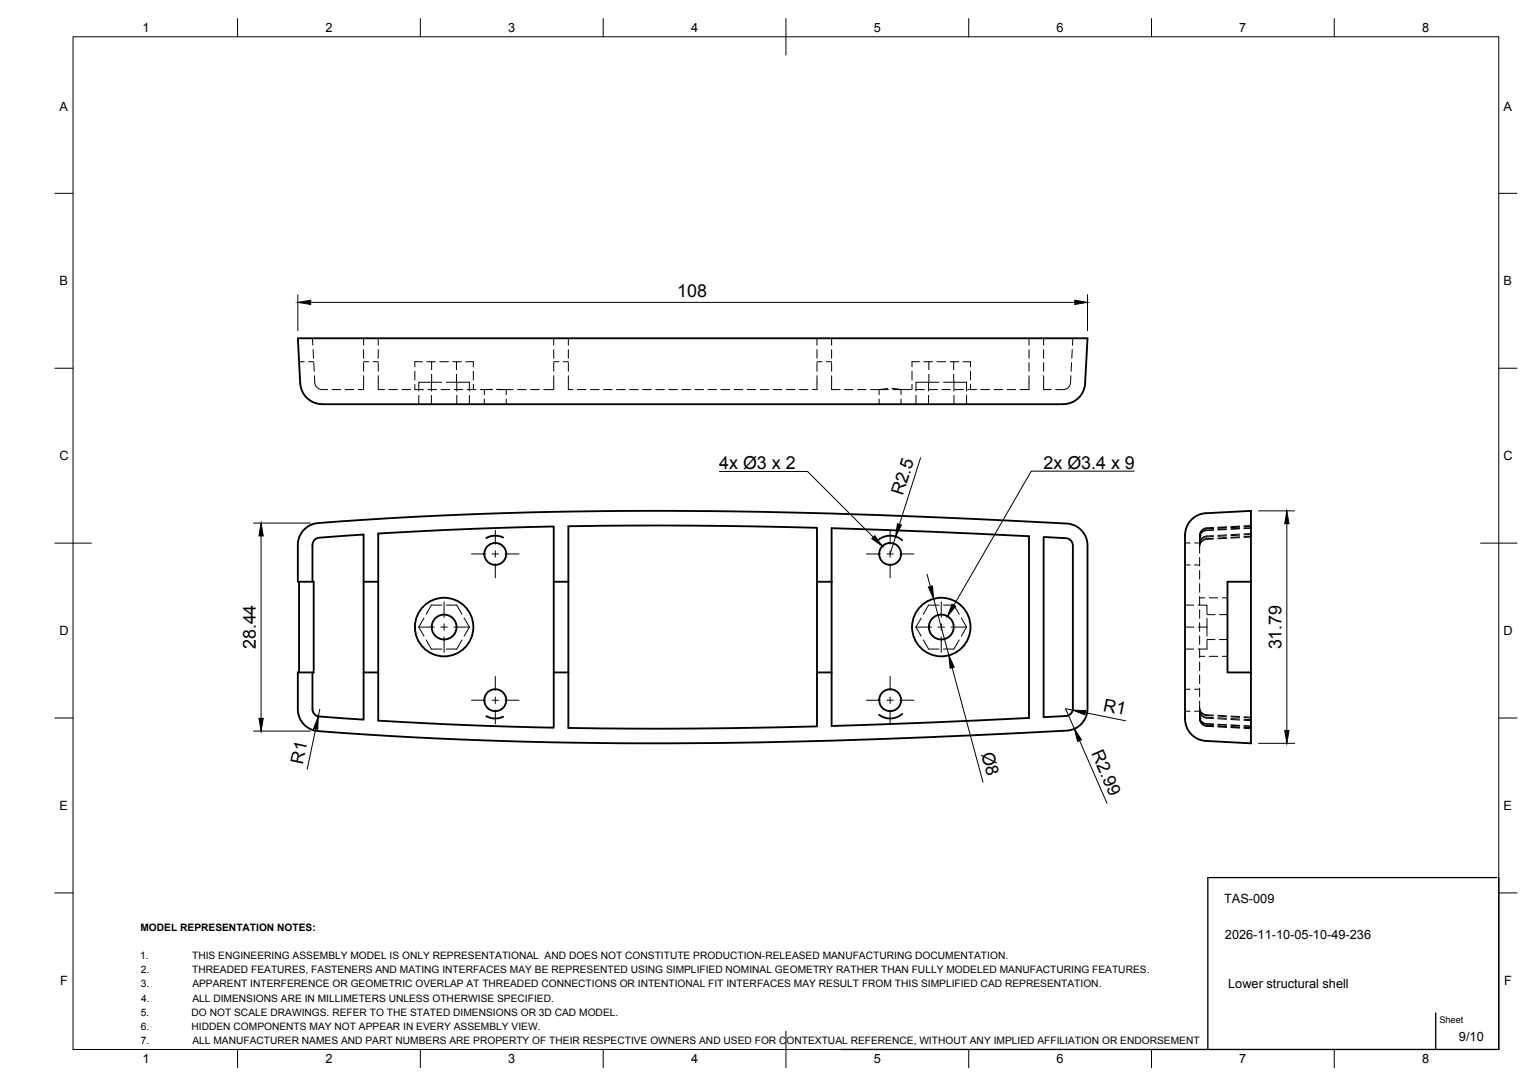
ISO-10303-21;
HEADER;
/* Generated by software containing ST-Developer
 * from STEP Tools, Inc. (www.steptools.com) 
 */

FILE_DESCRIPTION(
/* description */ (''),
/* implementation_level */ '2;1');

FILE_NAME(
/* name */ 'Lower structural shell.step',
/* time_stamp */ '2026-11-12T00:53:40-08:00',
/* author */ (''),
/* organization */ (''),
/* preprocessor_version */ 'ST-DEVELOPER v20.2',
/* originating_system */ 'Autodesk Translation Framework v15.17.0.0',
/* authorisation */ '');

FILE_SCHEMA (('AUTOMOTIVE_DESIGN { 1 0 10303 214 3 1 1 }'));
ENDSEC;

DATA;
#10=MECHANICAL_DESIGN_GEOMETRIC_PRESENTATION_REPRESENTATION('',(#576),#22129);
#84=SPHERICAL_SURFACE('',#9277,0.1);
#85=SPHERICAL_SURFACE('',#9280,0.0999999999999998);
#86=SPHERICAL_SURFACE('',#9284,0.0999999999999993);
#87=SPHERICAL_SURFACE('',#9288,0.1);
#88=SPHERICAL_SURFACE('',#9293,0.3);
#89=SPHERICAL_SURFACE('',#9297,0.3);
#90=SPHERICAL_SURFACE('',#9301,0.299999999999999);
#91=SPHERICAL_SURFACE('',#9306,0.3);
#124=B_SPLINE_SURFACE_WITH_KNOTS('',3,3,((#14410,#14411,#14412,#14413),
(#14414,#14415,#14416,#14417),(#14418,#14419,#14420,#14421),(#14422,#14423,
#14424,#14425),(#14426,#14427,#14428,#14429)),.UNSPECIFIED.,.F.,.F.,.F.,
(4,1,4),(4,4),(0.,0.571428571428571,1.),(1.0454440030657,3.44967454744645),
 .UNSPECIFIED.);
#125=B_SPLINE_SURFACE_WITH_KNOTS('',3,3,((#14502,#14503,#14504,#14505),
(#14506,#14507,#14508,#14509),(#14510,#14511,#14512,#14513),(#14514,#14515,
#14516,#14517),(#14518,#14519,#14520,#14521)),.UNSPECIFIED.,.F.,.F.,.F.,
(4,1,4),(4,4),(0.,0.571428571428571,1.),(7.24519303641511,9.95046872158573),
 .UNSPECIFIED.);
#126=B_SPLINE_SURFACE_WITH_KNOTS('',3,3,((#15443,#15444,#15445,#15446),
(#15447,#15448,#15449,#15450),(#15451,#15452,#15453,#15454),(#15455,#15456,
#15457,#15458)),.UNSPECIFIED.,.F.,.F.,.F.,(4,4),(4,4),(0.0705535719740953,
0.323522444336189),(0.0117434863834119,0.684857763552191),.UNSPECIFIED.);
#127=B_SPLINE_SURFACE_WITH_KNOTS('',3,3,((#15463,#15464,#15465,#15466),
(#15467,#15468,#15469,#15470),(#15471,#15472,#15473,#15474),(#15475,#15476,
#15477,#15478)),.UNSPECIFIED.,.F.,.F.,.F.,(4,4),(4,4),(0.0262419052680539,
0.0545428296147404),(0.0121538053864343,0.684980602226481),
 .UNSPECIFIED.);
#128=B_SPLINE_SURFACE_WITH_KNOTS('',3,3,((#15488,#15489,#15490,#15491),
(#15492,#15493,#15494,#15495),(#15496,#15497,#15498,#15499),(#15500,#15501,
#15502,#15503),(#15504,#15505,#15506,#15507)),.UNSPECIFIED.,.F.,.F.,.F.,
(4,1,4),(4,4),(0.,0.571428571428571,1.),(0.752061768057538,3.45733745322815),
 .UNSPECIFIED.);
#129=B_SPLINE_SURFACE_WITH_KNOTS('',3,3,((#15508,#15509,#15510,#15511),
(#15512,#15513,#15514,#15515),(#15516,#15517,#15518,#15519),(#15520,#15521,
#15522,#15523),(#15524,#15525,#15526,#15527)),.UNSPECIFIED.,.F.,.F.,.F.,
(4,1,4),(4,4),(0.,0.571428571428571,1.),(0.283259008618247,0.557056952888827),
 .UNSPECIFIED.);
#130=B_SPLINE_SURFACE_WITH_KNOTS('',3,3,((#15541,#15542,#15543,#15544),
(#15545,#15546,#15547,#15548),(#15549,#15550,#15551,#15552),(#15553,#15554,
#15555,#15556)),.UNSPECIFIED.,.F.,.F.,.F.,(4,4),(4,4),(0.67647755566375,
0.929446428026011),(0.0117434863436937,0.684857763580381),.UNSPECIFIED.);
#131=B_SPLINE_SURFACE_WITH_KNOTS('',3,3,((#15557,#15558,#15559,#15560),
(#15561,#15562,#15563,#15564),(#15565,#15566,#15567,#15568),(#15569,#15570,
#15571,#15572)),.UNSPECIFIED.,.F.,.F.,.F.,(4,4),(4,4),(0.945457170385156,
0.973758094731946),(0.0121538053598088,0.684980602226481),.UNSPECIFIED.);
#132=B_SPLINE_SURFACE_WITH_KNOTS('',3,3,((#15656,#15657,#15658,#15659),
(#15660,#15661,#15662,#15663),(#15664,#15665,#15666,#15667),(#15668,#15669,
#15670,#15671)),.UNSPECIFIED.,.F.,.F.,.F.,(4,4),(4,4),(0.341142793678372,
0.658675488550287),(0.0116221239297273,0.684255166525269),.UNSPECIFIED.);
#133=B_SPLINE_SURFACE_WITH_KNOTS('',3,3,((#15676,#15677,#15678,#15679),
(#15680,#15681,#15682,#15683),(#15684,#15685,#15686,#15687),(#15688,#15689,
#15690,#15691),(#15692,#15693,#15694,#15695)),.UNSPECIFIED.,.F.,.F.,.F.,
(4,1,4),(4,4),(0.,0.571428571428571,1.),(3.65450559744172,7.0548588409572),
 .UNSPECIFIED.);
#134=B_SPLINE_SURFACE_WITH_KNOTS('',3,3,((#15705,#15706,#15707,#15708),
(#15709,#15710,#15711,#15712),(#15713,#15714,#15715,#15716),(#15717,#15718,
#15719,#15720),(#15721,#15722,#15723,#15724)),.UNSPECIFIED.,.F.,.F.,.F.,
(4,1,4),(4,4),(0.,0.571428571428571,1.),(3.64767164868607,7.04802489220155),
 .UNSPECIFIED.);
#135=B_SPLINE_SURFACE_WITH_KNOTS('',3,3,((#15729,#15730,#15731,#15732),
(#15733,#15734,#15735,#15736),(#15737,#15738,#15739,#15740),(#15741,#15742,
#15743,#15744)),.UNSPECIFIED.,.F.,.F.,.F.,(4,4),(4,4),(0.341324511449716,
0.658857206321627),(0.0116221214776208,0.684255166525269),.UNSPECIFIED.);
#136=B_SPLINE_SURFACE_WITH_KNOTS('',3,3,((#15789,#15790,#15791,#15792),
(#15793,#15794,#15795,#15796),(#15797,#15798,#15799,#15800),(#15801,#15802,
#15803,#15804)),.UNSPECIFIED.,.F.,.F.,.F.,(4,4),(4,4),(0.676316266718331,
0.901708040522105),(0.0117102006467275,0.68495201331719),.UNSPECIFIED.);
#137=B_SPLINE_SURFACE_WITH_KNOTS('',3,3,((#15809,#15810,#15811,#15812),
(#15813,#15814,#15815,#15816),(#15817,#15818,#15819,#15820),(#15821,#15822,
#15823,#15824),(#15825,#15826,#15827,#15828)),.UNSPECIFIED.,.F.,.F.,.F.,
(4,1,4),(4,4),(0.,0.571428571428571,1.),(7.25285594219682,9.65708648657758),
 .UNSPECIFIED.);
#138=B_SPLINE_SURFACE_WITH_KNOTS('',3,3,((#15838,#15839,#15840,#15841),
(#15842,#15843,#15844,#15845),(#15846,#15847,#15848,#15849),(#15850,#15851,
#15852,#15853)),.UNSPECIFIED.,.F.,.F.,.F.,(4,4),(4,4),(0.0982919594778951,
0.323683733281714),(0.0117102006467272,0.68495201331719),.UNSPECIFIED.);
#139=B_SPLINE_SURFACE_WITH_KNOTS('',3,3,((#15928,#15929,#15930,#15931),
(#15932,#15933,#15934,#15935),(#15936,#15937,#15938,#15939),(#15940,#15941,
#15942,#15943)),.UNSPECIFIED.,.F.,.F.,.F.,(4,4),(4,4),(0.917922863855343,
0.974411608827007),(0.0122403473423911,0.685344304754238),.UNSPECIFIED.);
#140=B_SPLINE_SURFACE_WITH_KNOTS('',3,3,((#15953,#15954,#15955,#15956),
(#15957,#15958,#15959,#15960),(#15961,#15962,#15963,#15964),(#15965,#15966,
#15967,#15968),(#15969,#15970,#15971,#15972)),.UNSPECIFIED.,.F.,.F.,.F.,
(4,1,4),(4,4),(0.,0.571428571428571,1.),(9.85085636625011,10.4271318523291),
 .UNSPECIFIED.);
#141=B_SPLINE_SURFACE_WITH_KNOTS('',3,3,((#15986,#15987,#15988,#15989),
(#15990,#15991,#15992,#15993),(#15994,#15995,#15996,#15997),(#15998,#15999,
#16000,#16001)),.UNSPECIFIED.,.F.,.F.,.F.,(4,4),(4,4),(0.025588391172993,
0.0820771361446569),(0.0122403473423911,0.685344304754238),
 .UNSPECIFIED.);
#142=B_SPLINE_SURFACE_WITH_KNOTS('',3,3,((#16011,#16012,#16013,#16014),
(#16015,#16016,#16017,#16018),(#16019,#16020,#16021,#16022),(#16023,#16024,
#16025,#16026),(#16027,#16028,#16029,#16030)),.UNSPECIFIED.,.F.,.F.,.F.,
(4,1,4),(4,4),(0.,0.571428571428571,1.),(0.27539863731415,0.851674123393175),
 .UNSPECIFIED.);
#143=B_SPLINE_SURFACE_WITH_KNOTS('',3,3,((#16044,#16045,#16046,#16047),
(#16048,#16049,#16050,#16051),(#16052,#16053,#16054,#16055),(#16056,#16057,
#16058,#16059),(#16060,#16061,#16062,#16063)),.UNSPECIFIED.,.F.,.F.,.F.,
(4,1,4),(4,4),(0.,0.571428571428571,1.),(0.00944995813270487,0.618489359031386),
 .UNSPECIFIED.);
#144=B_SPLINE_SURFACE_WITH_KNOTS('',3,3,((#16070,#16071,#16072,#16073),
(#16074,#16075,#16076,#16077),(#16078,#16079,#16080,#16081),(#16082,#16083,
#16084,#16085),(#16086,#16087,#16088,#16089)),.UNSPECIFIED.,.F.,.F.,.F.,
(4,1,4),(4,4),(0.,0.571428571428571,1.),(0.00908570715245136,0.618164468641375),
 .UNSPECIFIED.);
#145=B_SPLINE_SURFACE_WITH_KNOTS('',3,3,((#16094,#16095,#16096,#16097),
(#16098,#16099,#16100,#16101),(#16102,#16103,#16104,#16105),(#16106,#16107,
#16108,#16109),(#16110,#16111,#16112,#16113)),.UNSPECIFIED.,.F.,.F.,.F.,
(4,1,4),(4,4),(0.,0.571428571428571,1.),(0.0091183540525243,0.618164468641375),
 .UNSPECIFIED.);
#146=B_SPLINE_SURFACE_WITH_KNOTS('',3,3,((#16118,#16119,#16120,#16121),
(#16122,#16123,#16124,#16125),(#16126,#16127,#16128,#16129),(#16130,#16131,
#16132,#16133),(#16134,#16135,#16136,#16137)),.UNSPECIFIED.,.F.,.F.,.F.,
(4,1,4),(4,4),(0.,0.571428571428571,1.),(10.1454735367545,10.419271481025),
 .UNSPECIFIED.);
#147=B_SPLINE_SURFACE_WITH_KNOTS('',3,3,((#16138,#16139,#16140,#16141),
(#16142,#16143,#16144,#16145),(#16146,#16147,#16148,#16149),(#16150,#16151,
#16152,#16153),(#16154,#16155,#16156,#16157)),.UNSPECIFIED.,.F.,.F.,.F.,
(4,1,4),(4,4),(0.,0.571428571428571,1.),(0.0094045468285345,0.618489359031386),
 .UNSPECIFIED.);
#148=B_SPLINE_SURFACE_WITH_KNOTS('',3,3,((#16183,#16184,#16185,#16186),
(#16187,#16188,#16189,#16190),(#16191,#16192,#16193,#16194),(#16195,#16196,
#16197,#16198),(#16199,#16200,#16201,#16202)),.UNSPECIFIED.,.F.,.F.,.F.,
(4,1,4),(4,4),(0.,0.571428571428571,1.),(-0.00535061636073277,0.618489359031386),
 .UNSPECIFIED.);
#149=B_SPLINE_SURFACE_WITH_KNOTS('',3,3,((#16221,#16222,#16223,#16224,#16225),
(#16226,#16227,#16228,#16229,#16230),(#16231,#16232,#16233,#16234,#16235),
(#16236,#16237,#16238,#16239,#16240),(#16241,#16242,#16243,#16244,#16245)),
 .UNSPECIFIED.,.F.,.F.,.F.,(4,1,4),(4,1,4),(0.,0.571428571428571,1.),(0.283259008618247,
4.63063308449434,10.4271318523291),.UNSPECIFIED.);
#150=B_SPLINE_SURFACE_WITH_KNOTS('',3,3,((#16256,#16257,#16258,#16259),
(#16260,#16261,#16262,#16263),(#16264,#16265,#16266,#16267),(#16268,#16269,
#16270,#16271),(#16272,#16273,#16274,#16275)),.UNSPECIFIED.,.F.,.F.,.F.,
(4,1,4),(4,4),(0.,0.571428571428571,1.),(-0.00578978989683084,0.618164468641375),
 .UNSPECIFIED.);
#151=B_SPLINE_SURFACE_WITH_KNOTS('',3,3,((#16284,#16285,#16286,#16287),
(#16288,#16289,#16290,#16291),(#16292,#16293,#16294,#16295),(#16296,#16297,
#16298,#16299),(#16300,#16301,#16302,#16303)),.UNSPECIFIED.,.F.,.F.,.F.,
(4,1,4),(4,4),(0.,0.571428571428571,1.),(-0.00569189159989896,0.618164468641375),
 .UNSPECIFIED.);
#152=B_SPLINE_SURFACE_WITH_KNOTS('',3,3,((#16312,#16313,#16314,#16315,#16316),
(#16317,#16318,#16319,#16320,#16321),(#16322,#16323,#16324,#16325,#16326),
(#16327,#16328,#16329,#16330,#16331),(#16332,#16333,#16334,#16335,#16336)),
 .UNSPECIFIED.,.F.,.F.,.F.,(4,1,4),(4,1,4),(0.,0.571428571428571,1.),(0.27539863731415,
4.62277271319024,10.419271481025),.UNSPECIFIED.);
#153=B_SPLINE_SURFACE_WITH_KNOTS('',3,3,((#16347,#16348,#16349,#16350),
(#16351,#16352,#16353,#16354),(#16355,#16356,#16357,#16358),(#16359,#16360,
#16361,#16362),(#16363,#16364,#16365,#16366)),.UNSPECIFIED.,.F.,.F.,.F.,
(4,1,4),(4,4),(0.,0.571428571428571,1.),(-0.0054868135546625,0.618489359031386),
 .UNSPECIFIED.);
#154=B_SPLINE_SURFACE_WITH_KNOTS('',3,3,((#16375,#16376,#16377,#16378),
(#16379,#16380,#16381,#16382),(#16383,#16384,#16385,#16386),(#16387,#16388,
#16389,#16390)),.UNSPECIFIED.,.F.,.F.,.F.,(4,4),(4,4),(0.026239262514127,
0.974414173651419),(0.,0.685344304754238),.UNSPECIFIED.);
#155=B_SPLINE_SURFACE_WITH_KNOTS('',3,3,((#16393,#16394,#16395,#16396),
(#16397,#16398,#16399,#16400),(#16401,#16402,#16403,#16404),(#16405,#16406,
#16407,#16408)),.UNSPECIFIED.,.F.,.F.,.F.,(4,4),(4,4),(0.0255858263485814,
0.973760737485873),(0.,0.685344304754238),.UNSPECIFIED.);
#272=B_SPLINE_CURVE_WITH_KNOTS('',3,(#14309,#14310,#14311,#14312,#14313,
#14314,#14315,#14316,#14317,#14318,#14319,#14320,#14321,#14322,#14323,#14324,
#14325,#14326,#14327,#14328,#14329,#14330,#14331,#14332),.UNSPECIFIED.,
 .F.,.F.,(4,2,2,2,2,2,2,2,2,2,2,4),(-0.337265338267783,-0.250544943628509,
-0.208272806508042,-0.186542211788094,-0.176382978682897,-0.170925844043069,
-0.16639450677335,-0.161077381235501,-0.15182241135393,-0.115009181549223,
-0.030206004227969,0.),.UNSPECIFIED.);
#273=B_SPLINE_CURVE_WITH_KNOTS('',3,(#14337,#14338,#14339,#14340,#14341,
#14342,#14343,#14344,#14345,#14346,#14347,#14348,#14349,#14350,#14351,#14352,
#14353,#14354,#14355,#14356),.UNSPECIFIED.,.F.,.F.,(4,2,2,2,2,2,2,2,2,4),
(-0.240982594686416,-0.16829976149504,-0.141836598208813,-0.129116059226128,
-0.121962912034391,-0.115857591426886,-0.108506552485159,-0.0948769875819265,
-0.0364654790774683,0.),.UNSPECIFIED.);
#274=B_SPLINE_CURVE_WITH_KNOTS('',3,(#14361,#14362,#14363,#14364,#14365,
#14366,#14367,#14368,#14369,#14370,#14371,#14372,#14373,#14374,#14375,#14376,
#14377,#14378,#14379,#14380),.UNSPECIFIED.,.F.,.F.,(4,2,2,2,2,2,2,2,2,4),
(-0.240981214998207,-0.168303541671295,-0.141841407502325,-0.129121097580905,
-0.121968013294536,-0.115862708924237,-0.108511643765797,-0.0948818976588229,
-0.0364681276985956,0.),.UNSPECIFIED.);
#275=B_SPLINE_CURVE_WITH_KNOTS('',3,(#14385,#14386,#14387,#14388,#14389,
#14390,#14391,#14392,#14393,#14394,#14395,#14396,#14397,#14398,#14399,#14400,
#14401,#14402,#14403,#14404,#14405,#14406,#14407,#14408),.UNSPECIFIED.,
 .F.,.F.,(4,2,2,2,2,2,2,2,2,2,2,4),(-0.337269388373684,-0.250545316912909,
-0.208282401844766,-0.186554569827561,-0.176396213396297,-0.17093921790305,
-0.16640782243471,-0.161090427650893,-0.151834477986603,-0.115010808423941,
-0.0302102096065556,0.),.UNSPECIFIED.);
#276=B_SPLINE_CURVE_WITH_KNOTS('',3,(#14431,#14432,#14433,#14434),
 .UNSPECIFIED.,.F.,.F.,(4,4),(1.0454440030657,2.52465537163019),
 .UNSPECIFIED.);
#277=B_SPLINE_CURVE_WITH_KNOTS('',3,(#14436,#14437,#14438,#14439,#14440,
#14441,#14442,#14443,#14444,#14445,#14446,#14447,#14448,#14449,#14450,#14451,
#14452,#14453,#14454,#14455,#14456,#14457,#14458,#14459,#14460,#14461,#14462,
#14463),.UNSPECIFIED.,.F.,.F.,(4,3,3,3,3,3,3,3,3,4),(-0.152193408756968,
-0.128427023368412,-0.115107736263918,-0.0911810900745799,-0.0780377802127556,
-0.0652031397886901,-0.0414031558437525,-0.0389949527774582,-0.0152076153333754,
0.),.UNSPECIFIED.);
#278=B_SPLINE_CURVE_WITH_KNOTS('',3,(#14465,#14466,#14467,#14468),
 .UNSPECIFIED.,.F.,.F.,(4,4),(-3.44967454744645,-1.05170160817356),
 .UNSPECIFIED.);
#279=B_SPLINE_CURVE_WITH_KNOTS('',3,(#14470,#14471,#14472,#14473,#14474,
#14475,#14476,#14477,#14478,#14479,#14480,#14481,#14482,#14483,#14484,#14485,
#14486,#14487,#14488,#14489,#14490,#14491,#14492,#14493,#14494,#14495,#14496,
#14497),.UNSPECIFIED.,.F.,.F.,(4,3,3,3,3,3,3,3,3,4),(-0.152278960443096,
-0.128503570101575,-0.115218572146868,-0.09145408274965,-0.0870214650669139,
-0.0781562978024333,-0.0542566895399357,-0.03908030849237,-0.0153296112319379,
0.),.UNSPECIFIED.);
#280=B_SPLINE_CURVE_WITH_KNOTS('',3,(#14498,#14499,#14500,#14501),
 .UNSPECIFIED.,.F.,.F.,(4,4),(2.75501813708031,3.4476340663212),
 .UNSPECIFIED.);
#281=B_SPLINE_CURVE_WITH_KNOTS('',3,(#14523,#14524,#14525,#14526),
 .UNSPECIFIED.,.F.,.F.,(4,4),(7.24810383506675,7.89761558728778),
 .UNSPECIFIED.);
#282=B_SPLINE_CURVE_WITH_KNOTS('',3,(#14528,#14529,#14530,#14531,#14532,
#14533,#14534,#14535,#14536,#14537,#14538,#14539,#14540,#14541,#14542,#14543,
#14544,#14545,#14546,#14547,#14548,#14549,#14550,#14551,#14552,#14553,#14554,
#14555),.UNSPECIFIED.,.F.,.F.,(4,3,3,3,3,3,3,3,3,4),(-0.152278869104567,
-0.128548794904564,-0.115192257893812,-0.0912773536606376,-0.0781090575823055,
-0.0652724057916263,-0.0414819581560496,-0.0390493575290778,-0.015259721743698,
0.),.UNSPECIFIED.);
#283=B_SPLINE_CURVE_WITH_KNOTS('',3,(#14557,#14558,#14559,#14560),
 .UNSPECIFIED.,.F.,.F.,(4,4),(-9.94532343034734,-7.24519303641511),
 .UNSPECIFIED.);
#284=B_SPLINE_CURVE_WITH_KNOTS('',3,(#14562,#14563,#14564,#14565,#14566,
#14567,#14568,#14569,#14570,#14571,#14572,#14573,#14574,#14575,#14576,#14577,
#14578,#14579,#14580,#14581,#14582,#14583,#14584,#14585,#14586,#14587,#14588,
#14589),.UNSPECIFIED.,.F.,.F.,(4,3,3,3,3,3,3,3,3,4),(-0.152181623618259,
-0.128410404494075,-0.115248188224843,-0.0914746846046984,-0.0869904866333268,
-0.0783028696190655,-0.0543945376065823,-0.0391651209697638,-0.0153884182770307,
0.),.UNSPECIFIED.);
#285=B_SPLINE_CURVE_WITH_KNOTS('',3,(#14590,#14591,#14592,#14593),
 .UNSPECIFIED.,.F.,.F.,(4,4),(8.21380824320284,9.95046871680089),
 .UNSPECIFIED.);
#286=B_SPLINE_CURVE_WITH_KNOTS('',3,(#14596,#14597,#14598,#14599),
 .UNSPECIFIED.,.F.,.F.,(4,4),(2.80491490332713,3.45442665446657),
 .UNSPECIFIED.);
#287=B_SPLINE_CURVE_WITH_KNOTS('',3,(#14603,#14604,#14605,#14606),
 .UNSPECIFIED.,.F.,.F.,(4,4),(0.752061768057538,2.48872224644044),
 .UNSPECIFIED.);
#288=B_SPLINE_CURVE_WITH_KNOTS('',3,(#14814,#14815,#14816,#14817,#14818,
#14819),.UNSPECIFIED.,.F.,.F.,(4,2,4),(-0.606700505977711,-0.303383635264422,
-0.000339350725729326),.UNSPECIFIED.);
#289=B_SPLINE_CURVE_WITH_KNOTS('',3,(#14820,#14821,#14822,#14823,#14824,
#14825,#14826,#14827,#14828,#14829,#14830,#14831,#14832,#14833,#14834,#14835,
#14836,#14837,#14838,#14839,#14840,#14841,#14842,#14843,#14844,#14845,#14846,
#14847),.UNSPECIFIED.,.F.,.F.,(4,3,3,3,3,3,3,3,3,4),(-0.152173579228948,
-0.128423230539522,-0.115115104157663,-0.0911927259648815,-0.0780672068328041,
-0.0652082609452843,-0.0414117413801899,-0.0390174000215468,-0.0152300060615686,
0.),.UNSPECIFIED.);
#290=B_SPLINE_CURVE_WITH_KNOTS('',3,(#14848,#14849,#14850,#14851,#14852,
#14853),.UNSPECIFIED.,.F.,.F.,(4,2,4),(-0.606471894652381,-0.303383500305553,
-0.00011071898471493),.UNSPECIFIED.);
#291=B_SPLINE_CURVE_WITH_KNOTS('',3,(#14857,#14858,#14859,#14860,#14861,
#14862),.UNSPECIFIED.,.F.,.F.,(4,2,4),(-0.606240625011114,-0.303433113375332,
-0.00010938105916114),.UNSPECIFIED.);
#292=B_SPLINE_CURVE_WITH_KNOTS('',3,(#14864,#14865,#14866,#14867,#14868,
#14869,#14870,#14871,#14872,#14873,#14874,#14875,#14876,#14877,#14878,#14879,
#14880,#14881,#14882,#14883,#14884,#14885,#14886,#14887,#14888,#14889,#14890,
#14891),.UNSPECIFIED.,.F.,.F.,(4,3,3,3,3,3,3,3,3,4),(-0.152281454644235,
-0.128508102092242,-0.115234945630277,-0.0914677943501604,-0.0870276017853555,
-0.0781846052914712,-0.0542821334115454,-0.0390966859411886,-0.0153419673568312,
0.),.UNSPECIFIED.);
#293=B_SPLINE_CURVE_WITH_KNOTS('',3,(#14893,#14894,#14895,#14896,#14897,
#14898),.UNSPECIFIED.,.F.,.F.,(4,2,4),(-0.606758573154242,-0.303433157101101,
-0.000627306481538803),.UNSPECIFIED.);
#294=B_SPLINE_CURVE_WITH_KNOTS('',3,(#14904,#14905,#14906,#14907,#14908,
#14909),.UNSPECIFIED.,.F.,.F.,(4,2,4),(-0.60617382748,-0.303436117212405,
-7.2700296824213E-5),.UNSPECIFIED.);
#295=B_SPLINE_CURVE_WITH_KNOTS('',3,(#14911,#14912,#14913,#14914,#14915,
#14916,#14917,#14918,#14919,#14920,#14921,#14922,#14923,#14924,#14925,#14926,
#14927,#14928,#14929,#14930,#14931,#14932,#14933,#14934,#14935,#14936,#14937,
#14938),.UNSPECIFIED.,.F.,.F.,(4,3,3,3,3,3,3,3,3,4),(-0.152282154327755,
-0.128558036203745,-0.115201429639692,-0.0912891813973639,-0.0781219052297615,
-0.065279687589213,-0.0414913146723999,-0.0390591331507366,-0.0152683745546824,
0.),.UNSPECIFIED.);
#296=B_SPLINE_CURVE_WITH_KNOTS('',3,(#14942,#14943,#14944,#14945,#14946,
#14947,#14948,#14949,#14950,#14951,#14952,#14953,#14954,#14955,#14956,#14957,
#14958,#14959,#14960,#14961,#14962,#14963,#14964,#14965,#14966,#14967,#14968,
#14969),.UNSPECIFIED.,.F.,.F.,(4,3,3,3,3,3,3,3,3,4),(-0.152283066055976,
-0.128508717930245,-0.115216472798554,-0.091451700383826,-0.087022506454752,
-0.0781485278686168,-0.0542483994686567,-0.0390758108455304,-0.0153274175274101,
0.),.UNSPECIFIED.);
#297=B_SPLINE_CURVE_WITH_KNOTS('',3,(#14971,#14972,#14973,#14974,#14975,
#14976),.UNSPECIFIED.,.F.,.F.,(4,2,4),(-0.606800264911061,-0.303436147592132,
-0.000699137727853738),.UNSPECIFIED.);
#298=B_SPLINE_CURVE_WITH_KNOTS('',3,(#14981,#14982,#14983,#14984,#14985,
#14986),.UNSPECIFIED.,.F.,.F.,(4,2,4),(-0.606915279655722,-0.30363236403835,
-0.000516487074480598),.UNSPECIFIED.);
#299=B_SPLINE_CURVE_WITH_KNOTS('',3,(#14990,#14991,#14992,#14993,#14994,
#14995,#14996,#14997,#14998,#14999,#15000,#15001,#15002,#15003,#15004,#15005,
#15006,#15007,#15008,#15009,#15010,#15011,#15012,#15013,#15014,#15015,#15016,
#15017),.UNSPECIFIED.,.F.,.F.,(4,3,3,3,3,3,3,3,3,4),(-0.152205325335401,
-0.128433618138404,-0.115304790388008,-0.091527299141506,-0.0870178586418932,
-0.0783866443643876,-0.0544751548276533,-0.0392137310602028,-0.0154203878854647,
0.),.UNSPECIFIED.);
#300=B_SPLINE_CURVE_WITH_KNOTS('',3,(#15019,#15020,#15021,#15022,#15023,
#15024),.UNSPECIFIED.,.F.,.F.,(4,2,4),(-0.606752424187958,-0.303632696349781,
-0.000353591088346872),.UNSPECIFIED.);
#301=B_SPLINE_CURVE_WITH_KNOTS('',3,(#15030,#15031,#15032,#15033),
 .UNSPECIFIED.,.F.,.F.,(4,4),(0.0116023361771303,0.618489359031386),
 .UNSPECIFIED.);
#302=B_SPLINE_CURVE_WITH_KNOTS('',3,(#15037,#15038,#15039,#15040),
 .UNSPECIFIED.,.F.,.F.,(4,4),(-0.618489359031386,-0.01160233617713),
 .UNSPECIFIED.);
#303=B_SPLINE_CURVE_WITH_KNOTS('',3,(#15043,#15044,#15045,#15046),
 .UNSPECIFIED.,.F.,.F.,(4,4),(7.01593971618694,9.71770560667459),
 .UNSPECIFIED.);
#304=B_SPLINE_CURVE_WITH_KNOTS('',3,(#15047,#15048,#15049,#15050),
 .UNSPECIFIED.,.F.,.F.,(4,4),(0.505945342046796,3.20718651982575),
 .UNSPECIFIED.);
#305=B_SPLINE_CURVE_WITH_KNOTS('',3,(#15053,#15054,#15055,#15056,#15057,
#15058,#15059),.UNSPECIFIED.,.F.,.F.,(4,3,4),(3.40717417387402,5.11170895874517,
6.80746068626633),.UNSPECIFIED.);
#306=B_SPLINE_CURVE_WITH_KNOTS('',3,(#15062,#15063,#15064,#15065),
 .UNSPECIFIED.,.F.,.F.,(4,4),(7.00766573366377,9.41198845520559),
 .UNSPECIFIED.);
#307=B_SPLINE_CURVE_WITH_KNOTS('',3,(#15069,#15070,#15071,#15072),
 .UNSPECIFIED.,.F.,.F.,(4,4),(9.61248784142317,10.2217363065808),
 .UNSPECIFIED.);
#308=B_SPLINE_CURVE_WITH_KNOTS('',3,(#15073,#15074,#15075,#15076,#15077,
#15078,#15079,#15080,#15081,#15082,#15083,#15084,#15085,#15086,#15087,#15088,
#15089,#15090,#15091,#15092,#15093,#15094,#15095,#15096,#15097,#15098,#15099,
#15100),.UNSPECIFIED.,.F.,.F.,(4,3,3,3,3,3,3,3,3,4),(0.,0.0238103109064959,
0.0390781362249314,0.0628635086275546,0.0641230352384255,0.0780643700703951,
0.101962174814111,0.113803522271848,0.137549611554782,0.149564734365165),
 .UNSPECIFIED.);
#309=B_SPLINE_CURVE_WITH_KNOTS('',3,(#15104,#15105,#15106,#15107,#15108,
#15109,#15110,#15111,#15112,#15113,#15114,#15115,#15116,#15117,#15118,#15119,
#15120,#15121,#15122,#15123,#15124,#15125,#15126,#15127,#15128,#15129,#15130,
#15131,#15132,#15133,#15134),.UNSPECIFIED.,.F.,.F.,(4,3,3,3,3,3,3,3,3,3,
4),(0.,0.0535521515156599,0.107729685495911,0.117233338918226,0.171447998942947,
0.1923696899792,0.234191611538245,0.288659693466396,0.341410301570312,0.395549383747909,
0.448696573746633),.UNSPECIFIED.);
#310=B_SPLINE_CURVE_WITH_KNOTS('',3,(#15136,#15137,#15138,#15139),
 .UNSPECIFIED.,.F.,.F.,(4,4),(0.0255858263485814,0.973760737485873),
 .UNSPECIFIED.);
#311=B_SPLINE_CURVE_WITH_KNOTS('',3,(#15141,#15142,#15143,#15144,#15145,
#15146,#15147,#15148,#15149,#15150,#15151,#15152,#15153,#15154,#15155,#15156,
#15157,#15158,#15159,#15160,#15161,#15162,#15163,#15164,#15165,#15166,#15167,
#15168,#15169,#15170,#15171),.UNSPECIFIED.,.F.,.F.,(4,3,3,3,3,3,3,3,3,3,
4),(0.,0.0535144560117858,0.107726856902975,0.117300577410231,0.171517675930231,
0.195438847090422,0.234297456941738,0.289665153342662,0.345032849743585,
0.40043206955427,0.455831289364955),.UNSPECIFIED.);
#312=B_SPLINE_CURVE_WITH_KNOTS('',3,(#15175,#15176,#15177,#15178,#15179,
#15180,#15181,#15182,#15183,#15184,#15185,#15186,#15187,#15188,#15189,#15190,
#15191,#15192,#15193,#15194,#15195,#15196,#15197,#15198,#15199,#15200,#15201,
#15202,#15203,#15204,#15205),.UNSPECIFIED.,.F.,.F.,(4,3,3,3,3,3,3,3,3,3,
4),(0.,0.053505543180391,0.107714168832353,0.117253997025819,0.171473395203321,
0.195418854185489,0.234223199196375,0.289607016015183,0.344990832833991,
0.400409777473312,0.455828722112633),.UNSPECIFIED.);
#313=B_SPLINE_CURVE_WITH_KNOTS('',3,(#15207,#15208,#15209,#15210),
 .UNSPECIFIED.,.F.,.F.,(4,4),(0.0262392625141271,0.974414173651419),
 .UNSPECIFIED.);
#314=B_SPLINE_CURVE_WITH_KNOTS('',3,(#15212,#15213,#15214,#15215,#15216,
#15217,#15218,#15219,#15220,#15221,#15222,#15223,#15224,#15225,#15226,#15227,
#15228,#15229,#15230,#15231,#15232,#15233,#15234,#15235,#15236,#15237,#15238,
#15239,#15240,#15241,#15242),.UNSPECIFIED.,.F.,.F.,(4,3,3,3,3,3,3,3,3,3,
4),(0.,0.0535648734523888,0.107747221190676,0.117299947751206,0.171510987106922,
0.192397607227928,0.234296687348373,0.288768001369001,0.341469499352622,
0.395597672314973,0.448700135162036),.UNSPECIFIED.);
#315=B_SPLINE_CURVE_WITH_KNOTS('',3,(#15245,#15246,#15247,#15248,#15249,
#15250,#15251,#15252,#15253,#15254,#15255,#15256,#15257,#15258,#15259,#15260,
#15261,#15262,#15263,#15264,#15265,#15266,#15267,#15268,#15269),
 .UNSPECIFIED.,.F.,.F.,(4,3,3,3,3,3,3,3,4),(0.,0.0238141989470671,0.0391004231578824,
0.0641320992313133,0.0780996136084711,0.101998806889826,0.113823260594808,
0.137564745199532,0.149565921982294),.UNSPECIFIED.);
#316=B_SPLINE_CURVE_WITH_KNOTS('',3,(#15271,#15272,#15273,#15274),
 .UNSPECIFIED.,.F.,.F.,(4,4),(2.76692059912875E-5,0.609394470571143),
 .UNSPECIFIED.);
#317=B_SPLINE_CURVE_WITH_KNOTS('',3,(#15277,#15278,#15279,#15280),
 .UNSPECIFIED.,.F.,.F.,(4,4),(0.809932799154201,3.21472245120952),
 .UNSPECIFIED.);
#318=B_SPLINE_CURVE_WITH_KNOTS('',3,(#15283,#15284,#15285,#15286,#15287,
#15288,#15289),.UNSPECIFIED.,.F.,.F.,(4,3,4),(3.41496637450242,5.11093193409745,
6.81591321610411),.UNSPECIFIED.);
#319=B_SPLINE_CURVE_WITH_KNOTS('',3,(#15293,#15294,#15295,#15296),
 .UNSPECIFIED.,.F.,.F.,(4,4),(9.91798263530139,10.2237206759544),
 .UNSPECIFIED.);
#320=B_SPLINE_CURVE_WITH_KNOTS('',3,(#15298,#15299,#15300,#15301,#15302,
#15303,#15304,#15305,#15306,#15307,#15308,#15309,#15310,#15311,#15312,#15313,
#15314,#15315,#15316,#15317,#15318,#15319,#15320,#15321,#15322,#15323,#15324,
#15325),.UNSPECIFIED.,.F.,.F.,(4,3,3,3,3,3,3,3,3,4),(0.,0.023807020713713,
0.039085080816122,0.0628703378723092,0.0651394887354207,0.0780750047750988,
0.101981498769656,0.114997221725907,0.138748569029605,0.151942344104828),
 .UNSPECIFIED.);
#321=B_SPLINE_CURVE_WITH_KNOTS('',3,(#15329,#15330,#15331,#15332,#15333,
#15334,#15335,#15336,#15337,#15338,#15339,#15340,#15341,#15342,#15343,#15344,
#15345,#15346,#15347,#15348,#15349,#15350,#15351,#15352,#15353,#15354,#15355,
#15356),.UNSPECIFIED.,.F.,.F.,(4,3,3,3,3,3,3,3,3,4),(0.,0.0238098191818892,
0.0391006681981376,0.0628849269680955,0.0651459659463291,0.0780999162396042,
0.102007524384594,0.115011225379555,0.138759376430353,0.151943200125079),
 .UNSPECIFIED.);
#322=B_SPLINE_CURVE_WITH_KNOTS('',3,(#15358,#15359,#15360,#15361),
 .UNSPECIFIED.,.F.,.F.,(4,4),(2.85486020485948E-5,0.305707210239178),
 .UNSPECIFIED.);
#323=B_SPLINE_CURVE_WITH_KNOTS('',3,(#15371,#15372,#15373,#15374,#15375,
#15376),.UNSPECIFIED.,.F.,.F.,(4,2,4),(-0.606446248197249,-0.303383959626182,
-6.4365448350312E-5),.UNSPECIFIED.);
#324=B_SPLINE_CURVE_WITH_KNOTS('',3,(#15378,#15379,#15380,#15381,#15382,
#15383),.UNSPECIFIED.,.F.,.F.,(4,2,4),(-0.60675170080159,-0.303384112192838,
-0.000369837888147484),.UNSPECIFIED.);
#325=B_SPLINE_CURVE_WITH_KNOTS('',3,(#15385,#15386,#15387,#15388,#15389,
#15390,#15391,#15392,#15393,#15394,#15395,#15396,#15397,#15398,#15399,#15400,
#15401,#15402,#15403,#15404,#15405,#15406,#15407,#15408,#15409,#15410,#15411,
#15412),.UNSPECIFIED.,.F.,.F.,(4,3,3,3,3,3,3,3,3,4),(-0.152162866344201,
-0.128411131698784,-0.115108013904405,-0.0911850729173883,-0.0780642464630149,
-0.0652023242402653,-0.0414053499882389,-0.0390151293250392,-0.0152279490549848,
0.),.UNSPECIFIED.);
#326=B_SPLINE_CURVE_WITH_KNOTS('',3,(#15415,#15416,#15417,#15418,#15419,
#15420,#15421,#15422,#15423,#15424,#15425,#15426,#15427,#15428,#15429,#15430,
#15431,#15432,#15433,#15434,#15435,#15436,#15437,#15438,#15439,#15440,#15441,
#15442),.UNSPECIFIED.,.F.,.F.,(4,3,3,3,3,3,3,3,3,4),(-0.152171297476962,
-0.128400300768352,-0.115247520946962,-0.0914735511738372,-0.0869860114952295,
-0.0783112904282795,-0.0544025203706761,-0.0391699941254272,-0.015391764586027,
0.),.UNSPECIFIED.);
#327=B_SPLINE_CURVE_WITH_KNOTS('',3,(#15459,#15460,#15461,#15462),
 .UNSPECIFIED.,.F.,.F.,(4,4),(-3.45733745322815,-0.757207059295936),
 .UNSPECIFIED.);
#328=B_SPLINE_CURVE_WITH_KNOTS('',3,(#15480,#15481,#15482,#15483),
 .UNSPECIFIED.,.F.,.F.,(4,4),(-0.557056952888827,-0.283259008618247),
 .UNSPECIFIED.);
#329=B_SPLINE_CURVE_WITH_KNOTS('',3,(#15484,#15485,#15486,#15487),
 .UNSPECIFIED.,.F.,.F.,(4,4),(-0.618164468641375,-0.0110156167597059),
 .UNSPECIFIED.);
#330=B_SPLINE_CURVE_WITH_KNOTS('',3,(#15529,#15530,#15531,#15532),
 .UNSPECIFIED.,.F.,.F.,(4,4),(0.283259011433088,0.551788488929761),
 .UNSPECIFIED.);
#331=B_SPLINE_CURVE_WITH_KNOTS('',3,(#15536,#15537,#15538,#15539),
 .UNSPECIFIED.,.F.,.F.,(4,4),(10.1507419987596,10.419271481025),
 .UNSPECIFIED.);
#332=B_SPLINE_CURVE_WITH_KNOTS('',3,(#15574,#15575,#15576,#15577),
 .UNSPECIFIED.,.F.,.F.,(4,4),(0.0110156167597055,0.618164468641375),
 .UNSPECIFIED.);
#333=B_SPLINE_CURVE_WITH_KNOTS('',3,(#15578,#15579,#15580,#15581),
 .UNSPECIFIED.,.F.,.F.,(4,4),(-10.419271481025,-10.1454735367545),
 .UNSPECIFIED.);
#334=B_SPLINE_CURVE_WITH_KNOTS('',3,(#15584,#15585,#15586,#15587,#15588,
#15589),.UNSPECIFIED.,.F.,.F.,(4,2,4),(-0.606211482799139,-0.303431960476852,
-9.19895310989571E-5),.UNSPECIFIED.);
#335=B_SPLINE_CURVE_WITH_KNOTS('',3,(#15591,#15592,#15593,#15594,#15595,
#15596,#15597,#15598,#15599,#15600,#15601,#15602,#15603,#15604,#15605,#15606,
#15607,#15608,#15609,#15610,#15611,#15612,#15613,#15614,#15615,#15616,#15617,
#15618),.UNSPECIFIED.,.F.,.F.,(4,3,3,3,3,3,3,3,3,4),(-0.152283340966725,
-0.128554242174982,-0.115196092098682,-0.0912819860997417,-0.0781117853096875,
-0.0652755629514801,-0.0414857317972147,-0.039051434275634,-0.0152612146291672,
0.),.UNSPECIFIED.);
#336=B_SPLINE_CURVE_WITH_KNOTS('',3,(#15622,#15623,#15624,#15625,#15626,
#15627,#15628,#15629,#15630,#15631,#15632,#15633,#15634,#15635,#15636,#15637,
#15638,#15639,#15640,#15641,#15642,#15643,#15644,#15645,#15646,#15647,#15648,
#15649),.UNSPECIFIED.,.F.,.F.,(4,3,3,3,3,3,3,3,3,4),(-0.152285570909379,
-0.128511627155755,-0.115232904621082,-0.0914664612111958,-0.0870286654075453,
-0.0781769338106538,-0.0542752301960614,-0.039092246575741,-0.0153386136911565,
0.),.UNSPECIFIED.);
#337=B_SPLINE_CURVE_WITH_KNOTS('',3,(#15650,#15651,#15652,#15653,#15654,
#15655),.UNSPECIFIED.,.F.,.F.,(4,2,4),(-0.606773318344362,-0.303431998667662,
-0.000653802131222458),.UNSPECIFIED.);
#338=B_SPLINE_CURVE_WITH_KNOTS('',3,(#15672,#15673,#15674,#15675),
 .UNSPECIFIED.,.F.,.F.,(4,4),(-7.05313168653828,-3.6572084986735),
 .UNSPECIFIED.);
#339=B_SPLINE_CURVE_WITH_KNOTS('',3,(#15696,#15697,#15698,#15699),
 .UNSPECIFIED.,.F.,.F.,(4,4),(3.65450559744172,7.0548588409572),
 .UNSPECIFIED.);
#340=B_SPLINE_CURVE_WITH_KNOTS('',3,(#15701,#15702,#15703,#15704),
 .UNSPECIFIED.,.F.,.F.,(4,4),(3.64767164868607,7.04802489220155),
 .UNSPECIFIED.);
#341=B_SPLINE_CURVE_WITH_KNOTS('',3,(#15725,#15726,#15727,#15728),
 .UNSPECIFIED.,.F.,.F.,(4,4),(-7.04532199096977,-3.64939880310499),
 .UNSPECIFIED.);
#342=B_SPLINE_CURVE_WITH_KNOTS('',3,(#15747,#15748,#15749,#15750,#15751,
#15752),.UNSPECIFIED.,.F.,.F.,(4,2,4),(-0.606200453641641,-0.30343602424441,
-9.0120313562092E-5),.UNSPECIFIED.);
#343=B_SPLINE_CURVE_WITH_KNOTS('',3,(#15754,#15755,#15756,#15757,#15758,
#15759,#15760,#15761,#15762,#15763,#15764,#15765,#15766,#15767,#15768,#15769,
#15770,#15771,#15772,#15773,#15774,#15775,#15776,#15777,#15778,#15779,#15780,
#15781),.UNSPECIFIED.,.F.,.F.,(4,3,3,3,3,3,3,3,3,4),(-0.152277688086818,
-0.128551334178815,-0.115197577176818,-0.0912856014461669,-0.0781191417238373,
-0.0652765169533013,-0.0414883027365163,-0.0390570310290822,-0.0152653090895913,
0.),.UNSPECIFIED.);
#344=B_SPLINE_CURVE_WITH_KNOTS('',3,(#15783,#15784,#15785,#15786,#15787,
#15788),.UNSPECIFIED.,.F.,.F.,(4,2,4),(-0.60678286609787,-0.303436074842897,
-0.000672492961417026),.UNSPECIFIED.);
#345=B_SPLINE_CURVE_WITH_KNOTS('',3,(#15805,#15806,#15807,#15808),
 .UNSPECIFIED.,.F.,.F.,(4,4),(-9.65082888146972,-7.25285594219682),
 .UNSPECIFIED.);
#346=B_SPLINE_CURVE_WITH_KNOTS('',3,(#15829,#15830,#15831,#15832),
 .UNSPECIFIED.,.F.,.F.,(4,4),(7.25489642332205,7.94751235889625),
 .UNSPECIFIED.);
#347=B_SPLINE_CURVE_WITH_KNOTS('',3,(#15833,#15834,#15835,#15836),
 .UNSPECIFIED.,.F.,.F.,(4,4),(8.17787511801303,9.65708648657758),
 .UNSPECIFIED.);
#348=B_SPLINE_CURVE_WITH_KNOTS('',3,(#15856,#15857,#15858,#15859,#15860,
#15861),.UNSPECIFIED.,.F.,.F.,(4,2,4),(-0.607007797795788,-0.303636495504298,
-0.000571323176327465),.UNSPECIFIED.);
#349=B_SPLINE_CURVE_WITH_KNOTS('',3,(#15863,#15864,#15865,#15866,#15867,
#15868,#15869,#15870,#15871,#15872,#15873,#15874,#15875,#15876,#15877,#15878,
#15879,#15880,#15881,#15882,#15883,#15884,#15885,#15886,#15887,#15888,#15889,
#15890),.UNSPECIFIED.,.F.,.F.,(4,3,3,3,3,3,3,3,3,4),(-0.152184339020145,
-0.128410461444444,-0.115096394428865,-0.0911692948751363,-0.0780261759644403,
-0.0651939085034322,-0.0413932235702045,-0.0389860720679279,-0.0151971168406065,
0.),.UNSPECIFIED.);
#350=B_SPLINE_CURVE_WITH_KNOTS('',3,(#15894,#15895,#15896,#15897,#15898,
#15899,#15900,#15901,#15902,#15903,#15904,#15905,#15906,#15907,#15908,#15909,
#15910,#15911,#15912,#15913,#15914,#15915,#15916,#15917,#15918,#15919,#15920,
#15921),.UNSPECIFIED.,.F.,.F.,(4,3,3,3,3,3,3,3,3,4),(-0.15219777746951,
-0.128424216118147,-0.115318679085322,-0.0915406112613293,-0.0870190514838729,
-0.0784197287877601,-0.0545085386658457,-0.0392329067084975,-0.0154317870320417,
0.),.UNSPECIFIED.);
#351=B_SPLINE_CURVE_WITH_KNOTS('',3,(#15922,#15923,#15924,#15925,#15926,
#15927),.UNSPECIFIED.,.F.,.F.,(4,2,4),(-0.606706256981509,-0.303636876939173,
-0.00026974181288697),.UNSPECIFIED.);
#352=B_SPLINE_CURVE_WITH_KNOTS('',3,(#15945,#15946,#15947,#15948),
 .UNSPECIFIED.,.F.,.F.,(4,4),(0.0112334529114386,0.618489359031386),
 .UNSPECIFIED.);
#353=B_SPLINE_CURVE_WITH_KNOTS('',3,(#15949,#15950,#15951,#15952),
 .UNSPECIFIED.,.F.,.F.,(4,4),(-10.4271318523291,-9.85085636625011),
 .UNSPECIFIED.);
#354=B_SPLINE_CURVE_WITH_KNOTS('',3,(#15975,#15976,#15977,#15978),
 .UNSPECIFIED.,.F.,.F.,(4,4),(9.85750350611301,10.4271318523291),
 .UNSPECIFIED.);
#355=B_SPLINE_CURVE_WITH_KNOTS('',3,(#15982,#15983,#15984,#15985),
 .UNSPECIFIED.,.F.,.F.,(4,4),(0.27539863731415,0.845026983530265),
 .UNSPECIFIED.);
#356=B_SPLINE_CURVE_WITH_KNOTS('',3,(#16003,#16004,#16005,#16006),
 .UNSPECIFIED.,.F.,.F.,(4,4),(-0.851674123393175,-0.27539863731415),
 .UNSPECIFIED.);
#357=B_SPLINE_CURVE_WITH_KNOTS('',3,(#16007,#16008,#16009,#16010),
 .UNSPECIFIED.,.F.,.F.,(4,4),(-0.618489359031386,-0.0112334529114389),
 .UNSPECIFIED.);
#358=B_SPLINE_CURVE_WITH_KNOTS('',3,(#16090,#16091,#16092,#16093),
 .UNSPECIFIED.,.F.,.F.,(4,4),(0.0112755522169305,0.618164468641375),
 .UNSPECIFIED.);
#359=B_SPLINE_CURVE_WITH_KNOTS('',3,(#16114,#16115,#16116,#16117),
 .UNSPECIFIED.,.F.,.F.,(4,4),(-0.618164468641375,-0.0112755522169305),
 .UNSPECIFIED.);
#360=B_SPLINE_CURVE_WITH_KNOTS('',3,(#16203,#16204,#16205,#16206),
 .UNSPECIFIED.,.F.,.F.,(4,4),(5.55111512312578E-17,0.618489359031386),
 .UNSPECIFIED.);
#361=B_SPLINE_CURVE_WITH_KNOTS('',3,(#16207,#16208,#16209,#16210),
 .UNSPECIFIED.,.F.,.F.,(4,4),(-0.618489359031386,-0.00110654915602034),
 .UNSPECIFIED.);
#362=B_SPLINE_CURVE_WITH_KNOTS('',3,(#16246,#16247,#16248,#16249,#16250),
 .UNSPECIFIED.,.F.,.F.,(4,1,4),(-10.4271318523291,-4.63063308449434,-0.283259008618247),
 .UNSPECIFIED.);
#363=B_SPLINE_CURVE_WITH_KNOTS('',3,(#16251,#16252,#16253,#16254,#16255),
 .UNSPECIFIED.,.F.,.F.,(4,1,4),(0.283259011433087,4.63063308449434,10.4271318523291),
 .UNSPECIFIED.);
#364=B_SPLINE_CURVE_WITH_KNOTS('',3,(#16276,#16277,#16278,#16279),
 .UNSPECIFIED.,.F.,.F.,(4,4),(0.000779732613545348,0.618164468641375),
 .UNSPECIFIED.);
#365=B_SPLINE_CURVE_WITH_KNOTS('',3,(#16280,#16281,#16282,#16283),
 .UNSPECIFIED.,.F.,.F.,(4,4),(-0.618164468641375,-4.9439619065339E-17),
 .UNSPECIFIED.);
#366=B_SPLINE_CURVE_WITH_KNOTS('',3,(#16304,#16305,#16306,#16307),
 .UNSPECIFIED.,.F.,.F.,(4,4),(3.0964814046186E-16,0.618164468641375),
 .UNSPECIFIED.);
#367=B_SPLINE_CURVE_WITH_KNOTS('',3,(#16308,#16309,#16310,#16311),
 .UNSPECIFIED.,.F.,.F.,(4,4),(-0.618164468641375,-0.0007797326135453),
 .UNSPECIFIED.);
#368=B_SPLINE_CURVE_WITH_KNOTS('',3,(#16337,#16338,#16339,#16340,#16341),
 .UNSPECIFIED.,.F.,.F.,(4,1,4),(-10.419271481025,-4.62277271319024,-0.27539863731415),
 .UNSPECIFIED.);
#369=B_SPLINE_CURVE_WITH_KNOTS('',3,(#16342,#16343,#16344,#16345,#16346),
 .UNSPECIFIED.,.F.,.F.,(4,1,4),(0.27539863731415,4.62277271319024,10.419271481025),
 .UNSPECIFIED.);
#370=B_SPLINE_CURVE_WITH_KNOTS('',3,(#16367,#16368,#16369,#16370),
 .UNSPECIFIED.,.F.,.F.,(4,4),(0.00110654915602046,0.618489359031386),
 .UNSPECIFIED.);
#371=B_SPLINE_CURVE_WITH_KNOTS('',3,(#16371,#16372,#16373,#16374),
 .UNSPECIFIED.,.F.,.F.,(4,4),(-0.618489359031386,6.93889390390723E-18),
 .UNSPECIFIED.);
#558=SHAPE_REPRESENTATION_RELATIONSHIP('SRR','None',#22178,#567);
#567=ADVANCED_BREP_SHAPE_REPRESENTATION('',(#585),#22124);
#576=STYLED_ITEM('',(#22235),#585);
#585=MANIFOLD_SOLID_BREP('Body1',#8807);
#616=FACE_BOUND('',#1661,.T.);
#617=FACE_BOUND('',#1662,.T.);
#618=FACE_BOUND('',#1663,.T.);
#619=FACE_BOUND('',#1671,.T.);
#620=FACE_BOUND('',#1679,.T.);
#621=FACE_BOUND('',#1694,.T.);
#622=FACE_BOUND('',#1696,.T.);
#623=FACE_BOUND('',#1708,.T.);
#624=FACE_BOUND('',#1729,.T.);
#625=FACE_BOUND('',#1730,.T.);
#626=FACE_BOUND('',#1731,.T.);
#627=FACE_BOUND('',#1766,.T.);
#628=FACE_BOUND('',#1767,.T.);
#629=FACE_BOUND('',#1768,.T.);
#630=FACE_BOUND('',#1769,.T.);
#631=FACE_BOUND('',#1770,.T.);
#632=FACE_BOUND('',#1771,.T.);
#824=PLANE('',#9207);
#825=PLANE('',#9211);
#826=PLANE('',#9212);
#827=PLANE('',#9213);
#828=PLANE('',#9214);
#829=PLANE('',#9215);
#830=PLANE('',#9216);
#831=PLANE('',#9217);
#832=PLANE('',#9219);
#833=PLANE('',#9220);
#834=PLANE('',#9221);
#835=PLANE('',#9222);
#836=PLANE('',#9223);
#837=PLANE('',#9224);
#838=PLANE('',#9225);
#839=PLANE('',#9241);
#840=PLANE('',#9242);
#841=PLANE('',#9243);
#842=PLANE('',#9244);
#843=PLANE('',#9245);
#844=PLANE('',#9246);
#845=PLANE('',#9247);
#846=PLANE('',#9248);
#847=PLANE('',#9250);
#848=PLANE('',#9252);
#849=PLANE('',#9253);
#850=PLANE('',#9254);
#851=PLANE('',#9255);
#852=PLANE('',#9256);
#853=PLANE('',#9257);
#854=PLANE('',#9258);
#855=PLANE('',#9259);
#856=PLANE('',#9260);
#857=PLANE('',#9261);
#858=PLANE('',#9262);
#859=PLANE('',#9266);
#860=PLANE('',#9268);
#861=PLANE('',#9269);
#862=PLANE('',#9270);
#863=PLANE('',#9271);
#864=PLANE('',#9272);
#865=PLANE('',#9273);
#866=PLANE('',#9275);
#867=PLANE('',#9292);
#868=PLANE('',#9311);
#869=PLANE('',#9312);
#870=PLANE('',#9313);
#1145=FACE_OUTER_BOUND('',#1654,.T.);
#1146=FACE_OUTER_BOUND('',#1655,.T.);
#1147=FACE_OUTER_BOUND('',#1656,.T.);
#1148=FACE_OUTER_BOUND('',#1657,.T.);
#1149=FACE_OUTER_BOUND('',#1658,.T.);
#1150=FACE_OUTER_BOUND('',#1659,.T.);
#1151=FACE_OUTER_BOUND('',#1660,.T.);
#1152=FACE_OUTER_BOUND('',#1664,.T.);
#1153=FACE_OUTER_BOUND('',#1665,.T.);
#1154=FACE_OUTER_BOUND('',#1666,.T.);
#1155=FACE_OUTER_BOUND('',#1667,.T.);
#1156=FACE_OUTER_BOUND('',#1668,.T.);
#1157=FACE_OUTER_BOUND('',#1669,.T.);
#1158=FACE_OUTER_BOUND('',#1670,.T.);
#1159=FACE_OUTER_BOUND('',#1672,.T.);
#1160=FACE_OUTER_BOUND('',#1673,.T.);
#1161=FACE_OUTER_BOUND('',#1674,.T.);
#1162=FACE_OUTER_BOUND('',#1675,.T.);
#1163=FACE_OUTER_BOUND('',#1676,.T.);
#1164=FACE_OUTER_BOUND('',#1677,.T.);
#1165=FACE_OUTER_BOUND('',#1678,.T.);
#1166=FACE_OUTER_BOUND('',#1680,.T.);
#1167=FACE_OUTER_BOUND('',#1681,.T.);
#1168=FACE_OUTER_BOUND('',#1682,.T.);
#1169=FACE_OUTER_BOUND('',#1683,.T.);
#1170=FACE_OUTER_BOUND('',#1684,.T.);
#1171=FACE_OUTER_BOUND('',#1685,.T.);
#1172=FACE_OUTER_BOUND('',#1686,.T.);
#1173=FACE_OUTER_BOUND('',#1687,.T.);
#1174=FACE_OUTER_BOUND('',#1688,.T.);
#1175=FACE_OUTER_BOUND('',#1689,.T.);
#1176=FACE_OUTER_BOUND('',#1690,.T.);
#1177=FACE_OUTER_BOUND('',#1691,.T.);
#1178=FACE_OUTER_BOUND('',#1692,.T.);
#1179=FACE_OUTER_BOUND('',#1693,.T.);
#1180=FACE_OUTER_BOUND('',#1695,.T.);
#1181=FACE_OUTER_BOUND('',#1697,.T.);
#1182=FACE_OUTER_BOUND('',#1698,.T.);
#1183=FACE_OUTER_BOUND('',#1699,.T.);
#1184=FACE_OUTER_BOUND('',#1700,.T.);
#1185=FACE_OUTER_BOUND('',#1701,.T.);
#1186=FACE_OUTER_BOUND('',#1702,.T.);
#1187=FACE_OUTER_BOUND('',#1703,.T.);
#1188=FACE_OUTER_BOUND('',#1704,.T.);
#1189=FACE_OUTER_BOUND('',#1705,.T.);
#1190=FACE_OUTER_BOUND('',#1706,.T.);
#1191=FACE_OUTER_BOUND('',#1707,.T.);
#1192=FACE_OUTER_BOUND('',#1709,.T.);
#1193=FACE_OUTER_BOUND('',#1710,.T.);
#1194=FACE_OUTER_BOUND('',#1711,.T.);
#1195=FACE_OUTER_BOUND('',#1712,.T.);
#1196=FACE_OUTER_BOUND('',#1713,.T.);
#1197=FACE_OUTER_BOUND('',#1714,.T.);
#1198=FACE_OUTER_BOUND('',#1715,.T.);
#1199=FACE_OUTER_BOUND('',#1716,.T.);
#1200=FACE_OUTER_BOUND('',#1717,.T.);
#1201=FACE_OUTER_BOUND('',#1718,.T.);
#1202=FACE_OUTER_BOUND('',#1719,.T.);
#1203=FACE_OUTER_BOUND('',#1720,.T.);
#1204=FACE_OUTER_BOUND('',#1721,.T.);
#1205=FACE_OUTER_BOUND('',#1722,.T.);
#1206=FACE_OUTER_BOUND('',#1723,.T.);
#1207=FACE_OUTER_BOUND('',#1724,.T.);
#1208=FACE_OUTER_BOUND('',#1725,.T.);
#1209=FACE_OUTER_BOUND('',#1726,.T.);
#1210=FACE_OUTER_BOUND('',#1727,.T.);
#1211=FACE_OUTER_BOUND('',#1728,.T.);
#1212=FACE_OUTER_BOUND('',#1732,.T.);
#1213=FACE_OUTER_BOUND('',#1733,.T.);
#1214=FACE_OUTER_BOUND('',#1734,.T.);
#1215=FACE_OUTER_BOUND('',#1735,.T.);
#1216=FACE_OUTER_BOUND('',#1736,.T.);
#1217=FACE_OUTER_BOUND('',#1737,.T.);
#1218=FACE_OUTER_BOUND('',#1738,.T.);
#1219=FACE_OUTER_BOUND('',#1739,.T.);
#1220=FACE_OUTER_BOUND('',#1740,.T.);
#1221=FACE_OUTER_BOUND('',#1741,.T.);
#1222=FACE_OUTER_BOUND('',#1742,.T.);
#1223=FACE_OUTER_BOUND('',#1743,.T.);
#1224=FACE_OUTER_BOUND('',#1744,.T.);
#1225=FACE_OUTER_BOUND('',#1745,.T.);
#1226=FACE_OUTER_BOUND('',#1746,.T.);
#1227=FACE_OUTER_BOUND('',#1747,.T.);
#1228=FACE_OUTER_BOUND('',#1748,.T.);
#1229=FACE_OUTER_BOUND('',#1749,.T.);
#1230=FACE_OUTER_BOUND('',#1750,.T.);
#1231=FACE_OUTER_BOUND('',#1751,.T.);
#1232=FACE_OUTER_BOUND('',#1752,.T.);
#1233=FACE_OUTER_BOUND('',#1753,.T.);
#1234=FACE_OUTER_BOUND('',#1754,.T.);
#1235=FACE_OUTER_BOUND('',#1755,.T.);
#1236=FACE_OUTER_BOUND('',#1756,.T.);
#1237=FACE_OUTER_BOUND('',#1757,.T.);
#1238=FACE_OUTER_BOUND('',#1758,.T.);
#1239=FACE_OUTER_BOUND('',#1759,.T.);
#1240=FACE_OUTER_BOUND('',#1760,.T.);
#1241=FACE_OUTER_BOUND('',#1761,.T.);
#1242=FACE_OUTER_BOUND('',#1762,.T.);
#1243=FACE_OUTER_BOUND('',#1763,.T.);
#1244=FACE_OUTER_BOUND('',#1764,.T.);
#1245=FACE_OUTER_BOUND('',#1765,.T.);
#1246=FACE_OUTER_BOUND('',#1772,.T.);
#1247=FACE_OUTER_BOUND('',#1773,.T.);
#1654=EDGE_LOOP('',(#6954,#6955));
#1655=EDGE_LOOP('',(#6956,#6957));
#1656=EDGE_LOOP('',(#6958,#6959));
#1657=EDGE_LOOP('',(#6960,#6961));
#1658=EDGE_LOOP('',(#6962,#6963,#6964,#6965,#6966,#6967));
#1659=EDGE_LOOP('',(#6968,#6969,#6970,#6971,#6972,#6973));
#1660=EDGE_LOOP('',(#6974,#6975,#6976,#6977,#6978,#6979,#6980,#6981));
#1661=EDGE_LOOP('',(#6982));
#1662=EDGE_LOOP('',(#6983));
#1663=EDGE_LOOP('',(#6984));
#1664=EDGE_LOOP('',(#6985,#6986,#6987,#6988));
#1665=EDGE_LOOP('',(#6989,#6990,#6991,#6992));
#1666=EDGE_LOOP('',(#6993,#6994,#6995,#6996));
#1667=EDGE_LOOP('',(#6997,#6998,#6999,#7000));
#1668=EDGE_LOOP('',(#7001,#7002,#7003,#7004));
#1669=EDGE_LOOP('',(#7005,#7006,#7007,#7008));
#1670=EDGE_LOOP('',(#7009,#7010,#7011,#7012,#7013,#7014));
#1671=EDGE_LOOP('',(#7015));
#1672=EDGE_LOOP('',(#7016,#7017,#7018,#7019));
#1673=EDGE_LOOP('',(#7020,#7021,#7022,#7023));
#1674=EDGE_LOOP('',(#7024,#7025,#7026,#7027));
#1675=EDGE_LOOP('',(#7028,#7029,#7030,#7031));
#1676=EDGE_LOOP('',(#7032,#7033,#7034,#7035));
#1677=EDGE_LOOP('',(#7036,#7037,#7038,#7039));
#1678=EDGE_LOOP('',(#7040,#7041,#7042,#7043,#7044,#7045));
#1679=EDGE_LOOP('',(#7046));
#1680=EDGE_LOOP('',(#7047,#7048,#7049,#7050));
#1681=EDGE_LOOP('',(#7051,#7052,#7053,#7054));
#1682=EDGE_LOOP('',(#7055,#7056,#7057,#7058));
#1683=EDGE_LOOP('',(#7059,#7060,#7061,#7062));
#1684=EDGE_LOOP('',(#7063,#7064,#7065,#7066));
#1685=EDGE_LOOP('',(#7067,#7068,#7069,#7070));
#1686=EDGE_LOOP('',(#7071,#7072,#7073,#7074));
#1687=EDGE_LOOP('',(#7075,#7076,#7077,#7078));
#1688=EDGE_LOOP('',(#7079,#7080,#7081,#7082));
#1689=EDGE_LOOP('',(#7083,#7084,#7085,#7086));
#1690=EDGE_LOOP('',(#7087,#7088,#7089,#7090));
#1691=EDGE_LOOP('',(#7091,#7092,#7093,#7094));
#1692=EDGE_LOOP('',(#7095,#7096,#7097,#7098));
#1693=EDGE_LOOP('',(#7099));
#1694=EDGE_LOOP('',(#7100));
#1695=EDGE_LOOP('',(#7101));
#1696=EDGE_LOOP('',(#7102));
#1697=EDGE_LOOP('',(#7103,#7104,#7105,#7106));
#1698=EDGE_LOOP('',(#7107,#7108,#7109,#7110));
#1699=EDGE_LOOP('',(#7111,#7112,#7113,#7114));
#1700=EDGE_LOOP('',(#7115,#7116,#7117,#7118));
#1701=EDGE_LOOP('',(#7119,#7120,#7121,#7122));
#1702=EDGE_LOOP('',(#7123,#7124,#7125,#7126,#7127,#7128));
#1703=EDGE_LOOP('',(#7129,#7130,#7131,#7132,#7133,#7134,#7135,#7136,#7137,
#7138));
#1704=EDGE_LOOP('',(#7139,#7140,#7141,#7142,#7143,#7144,#7145,#7146,#7147,
#7148));
#1705=EDGE_LOOP('',(#7149,#7150,#7151,#7152,#7153,#7154,#7155,#7156,#7157,
#7158));
#1706=EDGE_LOOP('',(#7159,#7160,#7161,#7162,#7163,#7164,#7165,#7166));
#1707=EDGE_LOOP('',(#7167,#7168,#7169,#7170,#7171,#7172,#7173,#7174,#7175,
#7176,#7177,#7178,#7179,#7180,#7181,#7182,#7183,#7184,#7185,#7186,#7187,
#7188,#7189,#7190,#7191,#7192,#7193,#7194,#7195,#7196,#7197,#7198,#7199,
#7200,#7201,#7202,#7203,#7204,#7205,#7206,#7207,#7208));
#1708=EDGE_LOOP('',(#7209,#7210,#7211,#7212,#7213,#7214));
#1709=EDGE_LOOP('',(#7215,#7216,#7217,#7218));
#1710=EDGE_LOOP('',(#7219,#7220,#7221,#7222));
#1711=EDGE_LOOP('',(#7223,#7224,#7225,#7226,#7227,#7228));
#1712=EDGE_LOOP('',(#7229,#7230,#7231,#7232));
#1713=EDGE_LOOP('',(#7233,#7234,#7235,#7236));
#1714=EDGE_LOOP('',(#7237,#7238,#7239,#7240,#7241,#7242));
#1715=EDGE_LOOP('',(#7243,#7244,#7245,#7246));
#1716=EDGE_LOOP('',(#7247,#7248,#7249,#7250));
#1717=EDGE_LOOP('',(#7251,#7252,#7253,#7254));
#1718=EDGE_LOOP('',(#7255,#7256,#7257,#7258));
#1719=EDGE_LOOP('',(#7259,#7260,#7261,#7262,#7263,#7264,#7265,#7266,#7267,
#7268));
#1720=EDGE_LOOP('',(#7269,#7270,#7271,#7272));
#1721=EDGE_LOOP('',(#7273,#7274,#7275,#7276));
#1722=EDGE_LOOP('',(#7277,#7278,#7279,#7280));
#1723=EDGE_LOOP('',(#7281,#7282,#7283,#7284));
#1724=EDGE_LOOP('',(#7285,#7286,#7287,#7288));
#1725=EDGE_LOOP('',(#7289,#7290,#7291,#7292,#7293,#7294,#7295,#7296,#7297,
#7298));
#1726=EDGE_LOOP('',(#7299,#7300,#7301,#7302));
#1727=EDGE_LOOP('',(#7303,#7304,#7305,#7306,#7307,#7308));
#1728=EDGE_LOOP('',(#7309,#7310,#7311,#7312,#7313,#7314,#7315,#7316));
#1729=EDGE_LOOP('',(#7317));
#1730=EDGE_LOOP('',(#7318));
#1731=EDGE_LOOP('',(#7319));
#1732=EDGE_LOOP('',(#7320,#7321,#7322,#7323));
#1733=EDGE_LOOP('',(#7324,#7325,#7326,#7327,#7328,#7329,#7330,#7331,#7332,
#7333));
#1734=EDGE_LOOP('',(#7334,#7335,#7336,#7337));
#1735=EDGE_LOOP('',(#7338,#7339,#7340,#7341));
#1736=EDGE_LOOP('',(#7342,#7343,#7344,#7345));
#1737=EDGE_LOOP('',(#7346,#7347,#7348,#7349));
#1738=EDGE_LOOP('',(#7350,#7351,#7352,#7353));
#1739=EDGE_LOOP('',(#7354,#7355,#7356));
#1740=EDGE_LOOP('',(#7357,#7358,#7359));
#1741=EDGE_LOOP('',(#7360,#7361,#7362));
#1742=EDGE_LOOP('',(#7363,#7364,#7365,#7366));
#1743=EDGE_LOOP('',(#7367,#7368,#7369,#7370));
#1744=EDGE_LOOP('',(#7371,#7372,#7373));
#1745=EDGE_LOOP('',(#7374,#7375,#7376,#7377));
#1746=EDGE_LOOP('',(#7378,#7379,#7380,#7381));
#1747=EDGE_LOOP('',(#7382,#7383,#7384,#7385));
#1748=EDGE_LOOP('',(#7386,#7387,#7388,#7389));
#1749=EDGE_LOOP('',(#7390,#7391,#7392,#7393));
#1750=EDGE_LOOP('',(#7394,#7395,#7396,#7397));
#1751=EDGE_LOOP('',(#7398,#7399,#7400));
#1752=EDGE_LOOP('',(#7401,#7402,#7403));
#1753=EDGE_LOOP('',(#7404,#7405,#7406));
#1754=EDGE_LOOP('',(#7407,#7408,#7409,#7410));
#1755=EDGE_LOOP('',(#7411,#7412,#7413,#7414));
#1756=EDGE_LOOP('',(#7415,#7416,#7417));
#1757=EDGE_LOOP('',(#7418,#7419,#7420,#7421));
#1758=EDGE_LOOP('',(#7422,#7423,#7424,#7425));
#1759=EDGE_LOOP('',(#7426,#7427,#7428,#7429));
#1760=EDGE_LOOP('',(#7430,#7431,#7432,#7433));
#1761=EDGE_LOOP('',(#7434,#7435,#7436,#7437));
#1762=EDGE_LOOP('',(#7438,#7439,#7440,#7441));
#1763=EDGE_LOOP('',(#7442,#7443,#7444,#7445));
#1764=EDGE_LOOP('',(#7446,#7447,#7448,#7449,#7450,#7451,#7452,#7453));
#1765=EDGE_LOOP('',(#7454,#7455,#7456,#7457));
#1766=EDGE_LOOP('',(#7458,#7459,#7460,#7461,#7462,#7463));
#1767=EDGE_LOOP('',(#7464,#7465,#7466,#7467,#7468,#7469));
#1768=EDGE_LOOP('',(#7470));
#1769=EDGE_LOOP('',(#7471));
#1770=EDGE_LOOP('',(#7472));
#1771=EDGE_LOOP('',(#7473));
#1772=EDGE_LOOP('',(#7474,#7475,#7476,#7477));
#1773=EDGE_LOOP('',(#7478,#7479,#7480,#7481));
#2414=LINE('',#14600,#3144);
#2415=LINE('',#14602,#3145);
#2416=LINE('',#14616,#3146);
#2417=LINE('',#14618,#3147);
#2418=LINE('',#14620,#3148);
#2419=LINE('',#14621,#3149);
#2420=LINE('',#14624,#3150);
#2421=LINE('',#14626,#3151);
#2422=LINE('',#14627,#3152);
#2423=LINE('',#14630,#3153);
#2424=LINE('',#14632,#3154);
#2425=LINE('',#14633,#3155);
#2426=LINE('',#14636,#3156);
#2427=LINE('',#14638,#3157);
#2428=LINE('',#14639,#3158);
#2429=LINE('',#14642,#3159);
#2430=LINE('',#14644,#3160);
#2431=LINE('',#14645,#3161);
#2432=LINE('',#14647,#3162);
#2433=LINE('',#14648,#3163);
#2434=LINE('',#14655,#3164);
#2435=LINE('',#14657,#3165);
#2436=LINE('',#14659,#3166);
#2437=LINE('',#14660,#3167);
#2438=LINE('',#14663,#3168);
#2439=LINE('',#14665,#3169);
#2440=LINE('',#14666,#3170);
#2441=LINE('',#14669,#3171);
#2442=LINE('',#14671,#3172);
#2443=LINE('',#14672,#3173);
#2444=LINE('',#14675,#3174);
#2445=LINE('',#14677,#3175);
#2446=LINE('',#14678,#3176);
#2447=LINE('',#14681,#3177);
#2448=LINE('',#14683,#3178);
#2449=LINE('',#14684,#3179);
#2450=LINE('',#14686,#3180);
#2451=LINE('',#14687,#3181);
#2452=LINE('',#14694,#3182);
#2453=LINE('',#14699,#3183);
#2454=LINE('',#14705,#3184);
#2455=LINE('',#14710,#3185);
#2456=LINE('',#14713,#3186);
#2457=LINE('',#14717,#3187);
#2458=LINE('',#14722,#3188);
#2459=LINE('',#14724,#3189);
#2460=LINE('',#14726,#3190);
#2461=LINE('',#14727,#3191);
#2462=LINE('',#14731,#3192);
#2463=LINE('',#14733,#3193);
#2464=LINE('',#14735,#3194);
#2465=LINE('',#14736,#3195);
#2466=LINE('',#14740,#3196);
#2467=LINE('',#14742,#3197);
#2468=LINE('',#14744,#3198);
#2469=LINE('',#14745,#3199);
#2470=LINE('',#14749,#3200);
#2471=LINE('',#14751,#3201);
#2472=LINE('',#14753,#3202);
#2473=LINE('',#14754,#3203);
#2474=LINE('',#14758,#3204);
#2475=LINE('',#14760,#3205);
#2476=LINE('',#14762,#3206);
#2477=LINE('',#14763,#3207);
#2478=LINE('',#14767,#3208);
#2479=LINE('',#14769,#3209);
#2480=LINE('',#14771,#3210);
#2481=LINE('',#14772,#3211);
#2482=LINE('',#14776,#3212);
#2483=LINE('',#14778,#3213);
#2484=LINE('',#14780,#3214);
#2485=LINE('',#14781,#3215);
#2486=LINE('',#14789,#3216);
#2487=LINE('',#14790,#3217);
#2488=LINE('',#14792,#3218);
#2489=LINE('',#14793,#3219);
#2490=LINE('',#14795,#3220);
#2491=LINE('',#14796,#3221);
#2492=LINE('',#14799,#3222);
#2493=LINE('',#14801,#3223);
#2494=LINE('',#14802,#3224);
#2495=LINE('',#14805,#3225);
#2496=LINE('',#14807,#3226);
#2497=LINE('',#14808,#3227);
#2498=LINE('',#14812,#3228);
#2499=LINE('',#14856,#3229);
#2500=LINE('',#14899,#3230);
#2501=LINE('',#14902,#3231);
#2502=LINE('',#14940,#3232);
#2503=LINE('',#14977,#3233);
#2504=LINE('',#14980,#3234);
#2505=LINE('',#14988,#3235);
#2506=LINE('',#15025,#3236);
#2507=LINE('',#15028,#3237);
#2508=LINE('',#15035,#3238);
#2509=LINE('',#15041,#3239);
#2510=LINE('',#15052,#3240);
#2511=LINE('',#15061,#3241);
#2512=LINE('',#15067,#3242);
#2513=LINE('',#15102,#3243);
#2514=LINE('',#15173,#3244);
#2515=LINE('',#15243,#3245);
#2516=LINE('',#15275,#3246);
#2517=LINE('',#15281,#3247);
#2518=LINE('',#15290,#3248);
#2519=LINE('',#15327,#3249);
#2520=LINE('',#15362,#3250);
#2521=LINE('',#15364,#3251);
#2522=LINE('',#15368,#3252);
#2523=LINE('',#15414,#3253);
#2524=LINE('',#15540,#3254);
#2525=LINE('',#15620,#3255);
#2526=LINE('',#15782,#3256);
#2527=LINE('',#15892,#3257);
#2528=LINE('',#15981,#3258);
#2529=LINE('',#16069,#3259);
#2530=LINE('',#16181,#3260);
#2531=LINE('',#16182,#3261);
#2532=LINE('',#16219,#3262);
#2533=LINE('',#16220,#3263);
#3144=VECTOR('',#10576,1.);
#3145=VECTOR('',#10577,1.);
#3146=VECTOR('',#10586,1.);
#3147=VECTOR('',#10587,1.);
#3148=VECTOR('',#10588,1.);
#3149=VECTOR('',#10589,1.);
#3150=VECTOR('',#10592,1.);
#3151=VECTOR('',#10593,1.);
#3152=VECTOR('',#10594,1.);
#3153=VECTOR('',#10597,1.);
#3154=VECTOR('',#10598,1.);
#3155=VECTOR('',#10599,1.);
#3156=VECTOR('',#10602,1.);
#3157=VECTOR('',#10603,1.);
#3158=VECTOR('',#10604,1.);
#3159=VECTOR('',#10607,1.);
#3160=VECTOR('',#10608,1.);
#3161=VECTOR('',#10609,1.);
#3162=VECTOR('',#10612,1.);
#3163=VECTOR('',#10613,1.);
#3164=VECTOR('',#10620,1.);
#3165=VECTOR('',#10621,1.);
#3166=VECTOR('',#10622,1.);
#3167=VECTOR('',#10623,1.);
#3168=VECTOR('',#10626,1.);
#3169=VECTOR('',#10627,1.);
#3170=VECTOR('',#10628,1.);
#3171=VECTOR('',#10631,1.);
#3172=VECTOR('',#10632,1.);
#3173=VECTOR('',#10633,1.);
#3174=VECTOR('',#10636,1.);
#3175=VECTOR('',#10637,1.);
#3176=VECTOR('',#10638,1.);
#3177=VECTOR('',#10641,1.);
#3178=VECTOR('',#10642,1.);
#3179=VECTOR('',#10643,1.);
#3180=VECTOR('',#10646,1.);
#3181=VECTOR('',#10647,1.);
#3182=VECTOR('',#10656,0.15);
#3183=VECTOR('',#10661,0.15);
#3184=VECTOR('',#10668,0.15);
#3185=VECTOR('',#10675,0.15);
#3186=VECTOR('',#10678,0.17);
#3187=VECTOR('',#10683,0.17);
#3188=VECTOR('',#10688,1.);
#3189=VECTOR('',#10689,1.);
#3190=VECTOR('',#10690,1.);
#3191=VECTOR('',#10691,1.);
#3192=VECTOR('',#10694,1.);
#3193=VECTOR('',#10695,1.);
#3194=VECTOR('',#10696,1.);
#3195=VECTOR('',#10697,1.);
#3196=VECTOR('',#10700,1.);
#3197=VECTOR('',#10701,1.);
#3198=VECTOR('',#10702,1.);
#3199=VECTOR('',#10703,1.);
#3200=VECTOR('',#10706,1.);
#3201=VECTOR('',#10707,1.);
#3202=VECTOR('',#10708,1.);
#3203=VECTOR('',#10709,1.);
#3204=VECTOR('',#10712,1.);
#3205=VECTOR('',#10713,1.);
#3206=VECTOR('',#10714,1.);
#3207=VECTOR('',#10715,1.);
#3208=VECTOR('',#10718,1.);
#3209=VECTOR('',#10719,1.);
#3210=VECTOR('',#10720,1.);
#3211=VECTOR('',#10721,1.);
#3212=VECTOR('',#10724,1.);
#3213=VECTOR('',#10725,1.);
#3214=VECTOR('',#10726,1.);
#3215=VECTOR('',#10727,1.);
#3216=VECTOR('',#10738,1.);
#3217=VECTOR('',#10739,1.);
#3218=VECTOR('',#10742,1.);
#3219=VECTOR('',#10743,1.);
#3220=VECTOR('',#10746,1.);
#3221=VECTOR('',#10747,1.);
#3222=VECTOR('',#10750,1.);
#3223=VECTOR('',#10751,1.);
#3224=VECTOR('',#10752,1.);
#3225=VECTOR('',#10755,1.);
#3226=VECTOR('',#10756,1.);
#3227=VECTOR('',#10757,1.);
#3228=VECTOR('',#10760,1.);
#3229=VECTOR('',#10763,1.);
#3230=VECTOR('',#10764,1.);
#3231=VECTOR('',#10767,1.);
#3232=VECTOR('',#10768,1.);
#3233=VECTOR('',#10769,1.);
#3234=VECTOR('',#10772,1.);
#3235=VECTOR('',#10773,1.);
#3236=VECTOR('',#10774,1.);
#3237=VECTOR('',#10777,1.);
#3238=VECTOR('',#10778,1.);
#3239=VECTOR('',#10779,1.);
#3240=VECTOR('',#10782,1.);
#3241=VECTOR('',#10783,1.);
#3242=VECTOR('',#10784,1.);
#3243=VECTOR('',#10785,1.);
#3244=VECTOR('',#10786,1.);
#3245=VECTOR('',#10787,1.);
#3246=VECTOR('',#10788,1.);
#3247=VECTOR('',#10789,1.);
#3248=VECTOR('',#10790,1.);
#3249=VECTOR('',#10791,1.);
#3250=VECTOR('',#10792,1.);
#3251=VECTOR('',#10795,0.4);
#3252=VECTOR('',#10800,0.4);
#3253=VECTOR('',#10803,1.);
#3254=VECTOR('',#10808,1.);
#3255=VECTOR('',#10811,1.);
#3256=VECTOR('',#10816,1.);
#3257=VECTOR('',#10821,1.);
#3258=VECTOR('',#10826,1.);
#3259=VECTOR('',#10859,1.);
#3260=VECTOR('',#10888,1.);
#3261=VECTOR('',#10889,1.);
#3262=VECTOR('',#10900,1.);
#3263=VECTOR('',#10901,1.);
#3460=CIRCLE('',#9200,0.25);
#3461=CIRCLE('',#9202,0.25);
#3462=CIRCLE('',#9204,0.25);
#3463=CIRCLE('',#9206,0.25);
#3464=CIRCLE('',#9208,0.15);
#3465=CIRCLE('',#9209,0.15);
#3466=CIRCLE('',#9210,0.4);
#3467=CIRCLE('',#9218,0.17);
#3468=CIRCLE('',#9226,0.17);
#3469=CIRCLE('',#9228,0.15);
#3470=CIRCLE('',#9230,0.15);
#3471=CIRCLE('',#9231,0.15);
#3472=CIRCLE('',#9233,0.15);
#3473=CIRCLE('',#9234,0.15);
#3474=CIRCLE('',#9236,0.15);
#3475=CIRCLE('',#9238,0.17);
#3476=CIRCLE('',#9240,0.17);
#3477=CIRCLE('',#9249,0.4);
#3478=CIRCLE('',#9251,0.4);
#3479=CIRCLE('',#9265,0.4);
#3480=CIRCLE('',#9267,0.1);
#3481=CIRCLE('',#9274,0.0999999999999995);
#3482=CIRCLE('',#9276,0.1);
#3483=CIRCLE('',#9278,0.1);
#3484=CIRCLE('',#9279,0.1);
#3485=CIRCLE('',#9281,0.0999999999999999);
#3486=CIRCLE('',#9282,0.0999999999999998);
#3487=CIRCLE('',#9283,0.0999999999999998);
#3488=CIRCLE('',#9285,0.0999999999999994);
#3489=CIRCLE('',#9286,0.0999999999999993);
#3490=CIRCLE('',#9289,0.0999999999999999);
#3491=CIRCLE('',#9290,0.1);
#3492=CIRCLE('',#9294,0.3);
#3493=CIRCLE('',#9295,0.3);
#3494=CIRCLE('',#9296,0.3);
#3495=CIRCLE('',#9298,0.3);
#3496=CIRCLE('',#9299,0.3);
#3497=CIRCLE('',#9300,0.3);
#3498=CIRCLE('',#9302,0.3);
#3499=CIRCLE('',#9303,0.299999999999999);
#3500=CIRCLE('',#9304,0.3);
#3501=CIRCLE('',#9307,0.3);
#3502=CIRCLE('',#9308,0.3);
#3503=CIRCLE('',#9309,0.3);
#3976=VERTEX_POINT('',#14307);
#3977=VERTEX_POINT('',#14308);
#3978=VERTEX_POINT('',#14335);
#3979=VERTEX_POINT('',#14336);
#3980=VERTEX_POINT('',#14359);
#3981=VERTEX_POINT('',#14360);
#3982=VERTEX_POINT('',#14383);
#3983=VERTEX_POINT('',#14384);
#3984=VERTEX_POINT('',#14430);
#3985=VERTEX_POINT('',#14435);
#3986=VERTEX_POINT('',#14464);
#3987=VERTEX_POINT('',#14469);
#3988=VERTEX_POINT('',#14522);
#3989=VERTEX_POINT('',#14527);
#3990=VERTEX_POINT('',#14556);
#3991=VERTEX_POINT('',#14561);
#3992=VERTEX_POINT('',#14595);
#3993=VERTEX_POINT('',#14601);
#3994=VERTEX_POINT('',#14607);
#3995=VERTEX_POINT('',#14609);
#3996=VERTEX_POINT('',#14611);
#3997=VERTEX_POINT('',#14614);
#3998=VERTEX_POINT('',#14615);
#3999=VERTEX_POINT('',#14617);
#4000=VERTEX_POINT('',#14619);
#4001=VERTEX_POINT('',#14623);
#4002=VERTEX_POINT('',#14625);
#4003=VERTEX_POINT('',#14629);
#4004=VERTEX_POINT('',#14631);
#4005=VERTEX_POINT('',#14635);
#4006=VERTEX_POINT('',#14637);
#4007=VERTEX_POINT('',#14641);
#4008=VERTEX_POINT('',#14643);
#4009=VERTEX_POINT('',#14650);
#4010=VERTEX_POINT('',#14653);
#4011=VERTEX_POINT('',#14654);
#4012=VERTEX_POINT('',#14656);
#4013=VERTEX_POINT('',#14658);
#4014=VERTEX_POINT('',#14662);
#4015=VERTEX_POINT('',#14664);
#4016=VERTEX_POINT('',#14668);
#4017=VERTEX_POINT('',#14670);
#4018=VERTEX_POINT('',#14674);
#4019=VERTEX_POINT('',#14676);
#4020=VERTEX_POINT('',#14680);
#4021=VERTEX_POINT('',#14682);
#4022=VERTEX_POINT('',#14689);
#4023=VERTEX_POINT('',#14692);
#4024=VERTEX_POINT('',#14696);
#4025=VERTEX_POINT('',#14698);
#4026=VERTEX_POINT('',#14702);
#4027=VERTEX_POINT('',#14704);
#4028=VERTEX_POINT('',#14708);
#4029=VERTEX_POINT('',#14712);
#4030=VERTEX_POINT('',#14716);
#4031=VERTEX_POINT('',#14720);
#4032=VERTEX_POINT('',#14721);
#4033=VERTEX_POINT('',#14723);
#4034=VERTEX_POINT('',#14725);
#4035=VERTEX_POINT('',#14729);
#4036=VERTEX_POINT('',#14730);
#4037=VERTEX_POINT('',#14732);
#4038=VERTEX_POINT('',#14734);
#4039=VERTEX_POINT('',#14738);
#4040=VERTEX_POINT('',#14739);
#4041=VERTEX_POINT('',#14741);
#4042=VERTEX_POINT('',#14743);
#4043=VERTEX_POINT('',#14747);
#4044=VERTEX_POINT('',#14748);
#4045=VERTEX_POINT('',#14750);
#4046=VERTEX_POINT('',#14752);
#4047=VERTEX_POINT('',#14756);
#4048=VERTEX_POINT('',#14757);
#4049=VERTEX_POINT('',#14759);
#4050=VERTEX_POINT('',#14761);
#4051=VERTEX_POINT('',#14765);
#4052=VERTEX_POINT('',#14766);
#4053=VERTEX_POINT('',#14768);
#4054=VERTEX_POINT('',#14770);
#4055=VERTEX_POINT('',#14774);
#4056=VERTEX_POINT('',#14775);
#4057=VERTEX_POINT('',#14777);
#4058=VERTEX_POINT('',#14779);
#4059=VERTEX_POINT('',#14783);
#4060=VERTEX_POINT('',#14786);
#4061=VERTEX_POINT('',#14798);
#4062=VERTEX_POINT('',#14800);
#4063=VERTEX_POINT('',#14804);
#4064=VERTEX_POINT('',#14806);
#4065=VERTEX_POINT('',#14810);
#4066=VERTEX_POINT('',#14811);
#4067=VERTEX_POINT('',#14813);
#4068=VERTEX_POINT('',#14855);
#4069=VERTEX_POINT('',#14863);
#4070=VERTEX_POINT('',#14892);
#4071=VERTEX_POINT('',#14901);
#4072=VERTEX_POINT('',#14903);
#4073=VERTEX_POINT('',#14910);
#4074=VERTEX_POINT('',#14939);
#4075=VERTEX_POINT('',#14941);
#4076=VERTEX_POINT('',#14970);
#4077=VERTEX_POINT('',#14979);
#4078=VERTEX_POINT('',#14987);
#4079=VERTEX_POINT('',#14989);
#4080=VERTEX_POINT('',#15018);
#4081=VERTEX_POINT('',#15027);
#4082=VERTEX_POINT('',#15029);
#4083=VERTEX_POINT('',#15034);
#4084=VERTEX_POINT('',#15036);
#4085=VERTEX_POINT('',#15051);
#4086=VERTEX_POINT('',#15060);
#4087=VERTEX_POINT('',#15066);
#4088=VERTEX_POINT('',#15068);
#4089=VERTEX_POINT('',#15101);
#4090=VERTEX_POINT('',#15103);
#4091=VERTEX_POINT('',#15135);
#4092=VERTEX_POINT('',#15140);
#4093=VERTEX_POINT('',#15172);
#4094=VERTEX_POINT('',#15174);
#4095=VERTEX_POINT('',#15206);
#4096=VERTEX_POINT('',#15211);
#4097=VERTEX_POINT('',#15244);
#4098=VERTEX_POINT('',#15270);
#4099=VERTEX_POINT('',#15276);
#4100=VERTEX_POINT('',#15282);
#4101=VERTEX_POINT('',#15291);
#4102=VERTEX_POINT('',#15292);
#4103=VERTEX_POINT('',#15297);
#4104=VERTEX_POINT('',#15326);
#4105=VERTEX_POINT('',#15328);
#4106=VERTEX_POINT('',#15357);
#4107=VERTEX_POINT('',#15366);
#4108=VERTEX_POINT('',#15370);
#4109=VERTEX_POINT('',#15377);
#4110=VERTEX_POINT('',#15384);
#4111=VERTEX_POINT('',#15413);
#4112=VERTEX_POINT('',#15479);
#4113=VERTEX_POINT('',#15528);
#4114=VERTEX_POINT('',#15535);
#4115=VERTEX_POINT('',#15573);
#4116=VERTEX_POINT('',#15583);
#4117=VERTEX_POINT('',#15590);
#4118=VERTEX_POINT('',#15619);
#4119=VERTEX_POINT('',#15621);
#4120=VERTEX_POINT('',#15746);
#4121=VERTEX_POINT('',#15753);
#4122=VERTEX_POINT('',#15855);
#4123=VERTEX_POINT('',#15862);
#4124=VERTEX_POINT('',#15891);
#4125=VERTEX_POINT('',#15893);
#4126=VERTEX_POINT('',#15944);
#4127=VERTEX_POINT('',#15973);
#4128=VERTEX_POINT('',#15980);
#4129=VERTEX_POINT('',#16002);
#4130=VERTEX_POINT('',#16037);
#4131=VERTEX_POINT('',#16065);
#4132=VERTEX_POINT('',#16160);
#4133=VERTEX_POINT('',#16161);
#4134=VERTEX_POINT('',#16163);
#4135=VERTEX_POINT('',#16167);
#4136=VERTEX_POINT('',#16168);
#4137=VERTEX_POINT('',#16170);
#4138=VERTEX_POINT('',#16174);
#4139=VERTEX_POINT('',#16175);
#4140=VERTEX_POINT('',#16177);
#4141=VERTEX_POINT('',#16212);
#4142=VERTEX_POINT('',#16213);
#4143=VERTEX_POINT('',#16215);
#5030=EDGE_CURVE('',#3976,#3977,#272,.T.);
#5031=EDGE_CURVE('',#3976,#3977,#3460,.T.);
#5032=EDGE_CURVE('',#3978,#3979,#273,.T.);
#5033=EDGE_CURVE('',#3978,#3979,#3461,.T.);
#5034=EDGE_CURVE('',#3980,#3981,#274,.T.);
#5035=EDGE_CURVE('',#3980,#3981,#3462,.T.);
#5036=EDGE_CURVE('',#3982,#3983,#275,.T.);
#5037=EDGE_CURVE('',#3982,#3983,#3463,.T.);
#5038=EDGE_CURVE('',#3984,#3979,#276,.T.);
#5039=EDGE_CURVE('',#3984,#3985,#277,.T.);
#5040=EDGE_CURVE('',#3986,#3985,#278,.T.);
#5041=EDGE_CURVE('',#3986,#3987,#279,.T.);
#5042=EDGE_CURVE('',#3978,#3987,#280,.T.);
#5043=EDGE_CURVE('',#3988,#3983,#281,.T.);
#5044=EDGE_CURVE('',#3988,#3989,#282,.T.);
#5045=EDGE_CURVE('',#3990,#3989,#283,.T.);
#5046=EDGE_CURVE('',#3990,#3991,#284,.T.);
#5047=EDGE_CURVE('',#3982,#3991,#285,.T.);
#5048=EDGE_CURVE('',#3976,#3992,#286,.T.);
#5049=EDGE_CURVE('',#3992,#3988,#2414,.T.);
#5050=EDGE_CURVE('',#3991,#3993,#2415,.T.);
#5051=EDGE_CURVE('',#3993,#3977,#287,.T.);
#5052=EDGE_CURVE('',#3994,#3994,#3464,.T.);
#5053=EDGE_CURVE('',#3995,#3995,#3465,.T.);
#5054=EDGE_CURVE('',#3996,#3996,#3466,.T.);
#5055=EDGE_CURVE('',#3997,#3998,#2416,.T.);
#5056=EDGE_CURVE('',#3997,#3999,#2417,.T.);
#5057=EDGE_CURVE('',#3999,#4000,#2418,.T.);
#5058=EDGE_CURVE('',#3998,#4000,#2419,.T.);
#5059=EDGE_CURVE('',#4001,#3997,#2420,.T.);
#5060=EDGE_CURVE('',#4001,#4002,#2421,.T.);
#5061=EDGE_CURVE('',#4002,#3999,#2422,.T.);
#5062=EDGE_CURVE('',#4003,#4001,#2423,.T.);
#5063=EDGE_CURVE('',#4003,#4004,#2424,.T.);
#5064=EDGE_CURVE('',#4004,#4002,#2425,.T.);
#5065=EDGE_CURVE('',#4005,#4003,#2426,.T.);
#5066=EDGE_CURVE('',#4005,#4006,#2427,.T.);
#5067=EDGE_CURVE('',#4006,#4004,#2428,.T.);
#5068=EDGE_CURVE('',#4007,#4005,#2429,.T.);
#5069=EDGE_CURVE('',#4007,#4008,#2430,.T.);
#5070=EDGE_CURVE('',#4008,#4006,#2431,.T.);
#5071=EDGE_CURVE('',#3998,#4007,#2432,.T.);
#5072=EDGE_CURVE('',#4000,#4008,#2433,.T.);
#5073=EDGE_CURVE('',#4009,#4009,#3467,.T.);
#5074=EDGE_CURVE('',#4010,#4011,#2434,.T.);
#5075=EDGE_CURVE('',#4010,#4012,#2435,.T.);
#5076=EDGE_CURVE('',#4012,#4013,#2436,.T.);
#5077=EDGE_CURVE('',#4011,#4013,#2437,.T.);
#5078=EDGE_CURVE('',#4014,#4010,#2438,.T.);
#5079=EDGE_CURVE('',#4014,#4015,#2439,.T.);
#5080=EDGE_CURVE('',#4015,#4012,#2440,.T.);
#5081=EDGE_CURVE('',#4016,#4014,#2441,.T.);
#5082=EDGE_CURVE('',#4016,#4017,#2442,.T.);
#5083=EDGE_CURVE('',#4017,#4015,#2443,.T.);
#5084=EDGE_CURVE('',#4018,#4016,#2444,.T.);
#5085=EDGE_CURVE('',#4018,#4019,#2445,.T.);
#5086=EDGE_CURVE('',#4019,#4017,#2446,.T.);
#5087=EDGE_CURVE('',#4020,#4018,#2447,.T.);
#5088=EDGE_CURVE('',#4020,#4021,#2448,.T.);
#5089=EDGE_CURVE('',#4021,#4019,#2449,.T.);
#5090=EDGE_CURVE('',#4011,#4020,#2450,.T.);
#5091=EDGE_CURVE('',#4013,#4021,#2451,.T.);
#5092=EDGE_CURVE('',#4022,#4022,#3468,.T.);
#5093=EDGE_CURVE('',#4023,#4023,#3469,.T.);
#5094=EDGE_CURVE('',#4023,#3994,#2452,.T.);
#5095=EDGE_CURVE('',#4024,#4024,#3470,.T.);
#5096=EDGE_CURVE('',#4024,#4025,#2453,.T.);
#5097=EDGE_CURVE('',#4025,#4025,#3471,.T.);
#5098=EDGE_CURVE('',#4026,#4026,#3472,.T.);
#5099=EDGE_CURVE('',#4026,#4027,#2454,.T.);
#5100=EDGE_CURVE('',#4027,#4027,#3473,.T.);
#5101=EDGE_CURVE('',#4028,#4028,#3474,.T.);
#5102=EDGE_CURVE('',#4028,#3995,#2455,.T.);
#5103=EDGE_CURVE('',#4022,#4029,#2456,.T.);
#5104=EDGE_CURVE('',#4029,#4029,#3475,.T.);
#5105=EDGE_CURVE('',#4009,#4030,#2457,.T.);
#5106=EDGE_CURVE('',#4030,#4030,#3476,.T.);
#5107=EDGE_CURVE('',#4031,#4032,#2458,.T.);
#5108=EDGE_CURVE('',#4033,#4031,#2459,.T.);
#5109=EDGE_CURVE('',#4034,#4033,#2460,.T.);
#5110=EDGE_CURVE('',#4034,#4032,#2461,.T.);
#5111=EDGE_CURVE('',#4035,#4036,#2462,.T.);
#5112=EDGE_CURVE('',#4035,#4037,#2463,.T.);
#5113=EDGE_CURVE('',#4038,#4037,#2464,.T.);
#5114=EDGE_CURVE('',#4036,#4038,#2465,.T.);
#5115=EDGE_CURVE('',#4039,#4040,#2466,.T.);
#5116=EDGE_CURVE('',#4039,#4041,#2467,.T.);
#5117=EDGE_CURVE('',#4042,#4041,#2468,.T.);
#5118=EDGE_CURVE('',#4040,#4042,#2469,.T.);
#5119=EDGE_CURVE('',#4043,#4044,#2470,.T.);
#5120=EDGE_CURVE('',#4043,#4045,#2471,.T.);
#5121=EDGE_CURVE('',#4046,#4045,#2472,.T.);
#5122=EDGE_CURVE('',#4044,#4046,#2473,.T.);
#5123=EDGE_CURVE('',#4047,#4048,#2474,.T.);
#5124=EDGE_CURVE('',#4047,#4049,#2475,.T.);
#5125=EDGE_CURVE('',#4050,#4049,#2476,.T.);
#5126=EDGE_CURVE('',#4048,#4050,#2477,.T.);
#5127=EDGE_CURVE('',#4051,#4052,#2478,.T.);
#5128=EDGE_CURVE('',#4053,#4051,#2479,.T.);
#5129=EDGE_CURVE('',#4054,#4053,#2480,.T.);
#5130=EDGE_CURVE('',#4054,#4052,#2481,.T.);
#5131=EDGE_CURVE('',#4055,#4056,#2482,.T.);
#5132=EDGE_CURVE('',#4057,#4055,#2483,.T.);
#5133=EDGE_CURVE('',#4058,#4057,#2484,.T.);
#5134=EDGE_CURVE('',#4058,#4056,#2485,.T.);
#5135=EDGE_CURVE('',#4059,#4059,#3477,.T.);
#5136=EDGE_CURVE('',#4060,#4060,#3478,.T.);
#5137=EDGE_CURVE('',#4032,#4047,#2486,.T.);
#5138=EDGE_CURVE('',#4049,#4034,#2487,.T.);
#5139=EDGE_CURVE('',#4052,#4035,#2488,.T.);
#5140=EDGE_CURVE('',#4037,#4054,#2489,.T.);
#5141=EDGE_CURVE('',#4056,#4039,#2490,.T.);
#5142=EDGE_CURVE('',#4041,#4058,#2491,.T.);
#5143=EDGE_CURVE('',#4061,#4043,#2492,.T.);
#5144=EDGE_CURVE('',#4062,#4061,#2493,.T.);
#5145=EDGE_CURVE('',#4045,#4062,#2494,.T.);
#5146=EDGE_CURVE('',#4063,#4061,#2495,.T.);
#5147=EDGE_CURVE('',#4064,#4063,#2496,.T.);
#5148=EDGE_CURVE('',#4062,#4064,#2497,.T.);
#5149=EDGE_CURVE('',#4065,#4066,#2498,.T.);
#5150=EDGE_CURVE('',#4067,#4066,#288,.T.);
#5151=EDGE_CURVE('',#3993,#4067,#289,.T.);
#5152=EDGE_CURVE('',#4065,#3990,#290,.T.);
#5153=EDGE_CURVE('',#4064,#4068,#2499,.T.);
#5154=EDGE_CURVE('',#3989,#4068,#291,.T.);
#5155=EDGE_CURVE('',#4069,#3992,#292,.T.);
#5156=EDGE_CURVE('',#4070,#4069,#293,.T.);
#5157=EDGE_CURVE('',#4070,#4046,#2500,.T.);
#5158=EDGE_CURVE('',#4057,#4071,#2501,.T.);
#5159=EDGE_CURVE('',#4072,#4071,#294,.T.);
#5160=EDGE_CURVE('',#4073,#4072,#295,.T.);
#5161=EDGE_CURVE('',#4074,#4073,#2502,.T.);
#5162=EDGE_CURVE('',#4075,#4074,#296,.T.);
#5163=EDGE_CURVE('',#4076,#4075,#297,.T.);
#5164=EDGE_CURVE('',#4076,#4042,#2503,.T.);
#5165=EDGE_CURVE('',#4053,#4077,#2504,.T.);
#5166=EDGE_CURVE('',#3985,#4077,#298,.T.);
#5167=EDGE_CURVE('',#4078,#3984,#2505,.T.);
#5168=EDGE_CURVE('',#4079,#4078,#299,.T.);
#5169=EDGE_CURVE('',#4080,#4079,#300,.T.);
#5170=EDGE_CURVE('',#4080,#4038,#2506,.T.);
#5171=EDGE_CURVE('',#4081,#4048,#2507,.T.);
#5172=EDGE_CURVE('',#4081,#4082,#301,.T.);
#5173=EDGE_CURVE('',#4082,#4083,#2508,.T.);
#5174=EDGE_CURVE('',#4083,#4084,#302,.T.);
#5175=EDGE_CURVE('',#4031,#4084,#2509,.T.);
#5176=EDGE_CURVE('',#4070,#4066,#303,.T.);
#5177=EDGE_CURVE('',#4065,#4068,#304,.T.);
#5178=EDGE_CURVE('',#4085,#4063,#2510,.T.);
#5179=EDGE_CURVE('',#4085,#4071,#305,.T.);
#5180=EDGE_CURVE('',#4086,#4055,#2511,.T.);
#5181=EDGE_CURVE('',#4086,#4077,#306,.T.);
#5182=EDGE_CURVE('',#4087,#4051,#2512,.T.);
#5183=EDGE_CURVE('',#4087,#4088,#307,.T.);
#5184=EDGE_CURVE('',#4088,#4081,#308,.T.);
#5185=EDGE_CURVE('',#4050,#4089,#2513,.T.);
#5186=EDGE_CURVE('',#4090,#4089,#309,.T.);
#5187=EDGE_CURVE('',#4090,#4091,#310,.T.);
#5188=EDGE_CURVE('',#4092,#4091,#311,.T.);
#5189=EDGE_CURVE('',#4092,#4093,#2514,.T.);
#5190=EDGE_CURVE('',#4094,#4093,#312,.T.);
#5191=EDGE_CURVE('',#4094,#4095,#313,.T.);
#5192=EDGE_CURVE('',#4096,#4095,#314,.T.);
#5193=EDGE_CURVE('',#4096,#4033,#2515,.T.);
#5194=EDGE_CURVE('',#4084,#4097,#315,.T.);
#5195=EDGE_CURVE('',#4097,#4098,#316,.T.);
#5196=EDGE_CURVE('',#4036,#4098,#2516,.T.);
#5197=EDGE_CURVE('',#4080,#4099,#317,.T.);
#5198=EDGE_CURVE('',#4040,#4099,#2517,.T.);
#5199=EDGE_CURVE('',#4076,#4100,#318,.T.);
#5200=EDGE_CURVE('',#4044,#4100,#2518,.T.);
#5201=EDGE_CURVE('',#4101,#4102,#319,.T.);
#5202=EDGE_CURVE('',#4102,#4103,#320,.T.);
#5203=EDGE_CURVE('',#4103,#4104,#2519,.T.);
#5204=EDGE_CURVE('',#4104,#4105,#321,.T.);
#5205=EDGE_CURVE('',#4105,#4106,#322,.T.);
#5206=EDGE_CURVE('',#4101,#4106,#2520,.T.);
#5207=EDGE_CURVE('',#3996,#4060,#2521,.T.);
#5208=EDGE_CURVE('',#4107,#4107,#3479,.T.);
#5209=EDGE_CURVE('',#4107,#4059,#2522,.T.);
#5210=EDGE_CURVE('',#4101,#4108,#323,.T.);
#5211=EDGE_CURVE('',#4109,#4106,#324,.T.);
#5212=EDGE_CURVE('',#4110,#4109,#325,.T.);
#5213=EDGE_CURVE('',#4111,#4110,#2523,.T.);
#5214=EDGE_CURVE('',#4108,#4111,#326,.T.);
#5215=EDGE_CURVE('',#4069,#4067,#327,.T.);
#5216=EDGE_CURVE('',#4108,#4112,#328,.T.);
#5217=EDGE_CURVE('',#4112,#4102,#329,.T.);
#5218=EDGE_CURVE('',#4113,#4111,#330,.T.);
#5219=EDGE_CURVE('',#4112,#4113,#3480,.F.);
#5220=EDGE_CURVE('',#4110,#4114,#331,.T.);
#5221=EDGE_CURVE('',#4114,#4113,#2524,.T.);
#5222=EDGE_CURVE('',#4105,#4115,#332,.T.);
#5223=EDGE_CURVE('',#4115,#4109,#333,.T.);
#5224=EDGE_CURVE('',#4116,#4100,#334,.T.);
#5225=EDGE_CURVE('',#4117,#4116,#335,.T.);
#5226=EDGE_CURVE('',#4118,#4117,#2525,.T.);
#5227=EDGE_CURVE('',#4119,#4118,#336,.T.);
#5228=EDGE_CURVE('',#4085,#4119,#337,.T.);
#5229=EDGE_CURVE('',#4075,#4116,#338,.T.);
#5230=EDGE_CURVE('',#4117,#4074,#339,.T.);
#5231=EDGE_CURVE('',#4073,#4118,#340,.T.);
#5232=EDGE_CURVE('',#4119,#4072,#341,.T.);
#5233=EDGE_CURVE('',#4120,#4099,#342,.T.);
#5234=EDGE_CURVE('',#4121,#4120,#343,.T.);
#5235=EDGE_CURVE('',#3987,#4121,#2526,.T.);
#5236=EDGE_CURVE('',#4086,#3986,#344,.T.);
#5237=EDGE_CURVE('',#4079,#4120,#345,.T.);
#5238=EDGE_CURVE('',#4121,#3981,#346,.T.);
#5239=EDGE_CURVE('',#3980,#4078,#347,.T.);
#5240=EDGE_CURVE('',#4122,#4098,#348,.T.);
#5241=EDGE_CURVE('',#4123,#4122,#349,.T.);
#5242=EDGE_CURVE('',#4124,#4123,#2527,.T.);
#5243=EDGE_CURVE('',#4125,#4124,#350,.T.);
#5244=EDGE_CURVE('',#4087,#4125,#351,.T.);
#5245=EDGE_CURVE('',#4097,#4126,#352,.T.);
#5246=EDGE_CURVE('',#4126,#4122,#353,.T.);
#5247=EDGE_CURVE('',#4127,#4126,#3481,.F.);
#5248=EDGE_CURVE('',#4123,#4127,#354,.T.);
#5249=EDGE_CURVE('',#4127,#4128,#2528,.T.);
#5250=EDGE_CURVE('',#4128,#4124,#355,.T.);
#5251=EDGE_CURVE('',#4125,#4129,#356,.T.);
#5252=EDGE_CURVE('',#4129,#4088,#357,.T.);
#5253=EDGE_CURVE('',#4129,#4128,#3482,.F.);
#5254=EDGE_CURVE('',#4128,#4082,#3483,.F.);
#5255=EDGE_CURVE('',#4082,#4129,#3484,.F.);
#5256=EDGE_CURVE('',#4114,#4115,#3485,.F.);
#5257=EDGE_CURVE('',#4115,#4130,#3486,.F.);
#5258=EDGE_CURVE('',#4130,#4114,#3487,.F.);
#5259=EDGE_CURVE('',#4126,#4083,#3488,.F.);
#5260=EDGE_CURVE('',#4083,#4127,#3489,.F.);
#5261=EDGE_CURVE('',#4131,#4112,#3490,.F.);
#5262=EDGE_CURVE('',#4113,#4131,#3491,.F.);
#5263=EDGE_CURVE('',#4131,#4130,#2529,.T.);
#5264=EDGE_CURVE('',#4103,#4131,#358,.T.);
#5265=EDGE_CURVE('',#4130,#4104,#359,.T.);
#5266=EDGE_CURVE('',#4132,#4133,#3492,.F.);
#5267=EDGE_CURVE('',#4134,#4132,#3493,.F.);
#5268=EDGE_CURVE('',#4133,#4134,#3494,.F.);
#5269=EDGE_CURVE('',#4135,#4136,#3495,.F.);
#5270=EDGE_CURVE('',#4137,#4135,#3496,.F.);
#5271=EDGE_CURVE('',#4136,#4137,#3497,.F.);
#5272=EDGE_CURVE('',#4138,#4139,#3498,.F.);
#5273=EDGE_CURVE('',#4140,#4138,#3499,.F.);
#5274=EDGE_CURVE('',#4139,#4140,#3500,.F.);
#5275=EDGE_CURVE('',#4133,#4140,#2530,.T.);
#5276=EDGE_CURVE('',#4138,#4132,#2531,.T.);
#5277=EDGE_CURVE('',#4095,#4139,#360,.T.);
#5278=EDGE_CURVE('',#4140,#4096,#361,.T.);
#5279=EDGE_CURVE('',#4141,#4142,#3501,.F.);
#5280=EDGE_CURVE('',#4143,#4141,#3502,.F.);
#5281=EDGE_CURVE('',#4142,#4143,#3503,.F.);
#5282=EDGE_CURVE('',#4141,#4137,#2532,.T.);
#5283=EDGE_CURVE('',#4135,#4143,#2533,.T.);
#5284=EDGE_CURVE('',#4139,#4142,#362,.T.);
#5285=EDGE_CURVE('',#4143,#4138,#363,.T.);
#5286=EDGE_CURVE('',#4093,#4141,#364,.T.);
#5287=EDGE_CURVE('',#4142,#4094,#365,.T.);
#5288=EDGE_CURVE('',#4091,#4136,#366,.T.);
#5289=EDGE_CURVE('',#4137,#4092,#367,.T.);
#5290=EDGE_CURVE('',#4136,#4134,#368,.T.);
#5291=EDGE_CURVE('',#4132,#4135,#369,.T.);
#5292=EDGE_CURVE('',#4089,#4133,#370,.T.);
#5293=EDGE_CURVE('',#4134,#4090,#371,.T.);
#6954=ORIENTED_EDGE('',*,*,#5030,.F.);
#6955=ORIENTED_EDGE('',*,*,#5031,.T.);
#6956=ORIENTED_EDGE('',*,*,#5032,.F.);
#6957=ORIENTED_EDGE('',*,*,#5033,.T.);
#6958=ORIENTED_EDGE('',*,*,#5034,.F.);
#6959=ORIENTED_EDGE('',*,*,#5035,.T.);
#6960=ORIENTED_EDGE('',*,*,#5036,.F.);
#6961=ORIENTED_EDGE('',*,*,#5037,.T.);
#6962=ORIENTED_EDGE('',*,*,#5032,.T.);
#6963=ORIENTED_EDGE('',*,*,#5038,.F.);
#6964=ORIENTED_EDGE('',*,*,#5039,.T.);
#6965=ORIENTED_EDGE('',*,*,#5040,.F.);
#6966=ORIENTED_EDGE('',*,*,#5041,.T.);
#6967=ORIENTED_EDGE('',*,*,#5042,.F.);
#6968=ORIENTED_EDGE('',*,*,#5036,.T.);
#6969=ORIENTED_EDGE('',*,*,#5043,.F.);
#6970=ORIENTED_EDGE('',*,*,#5044,.T.);
#6971=ORIENTED_EDGE('',*,*,#5045,.F.);
#6972=ORIENTED_EDGE('',*,*,#5046,.T.);
#6973=ORIENTED_EDGE('',*,*,#5047,.F.);
#6974=ORIENTED_EDGE('',*,*,#5048,.T.);
#6975=ORIENTED_EDGE('',*,*,#5049,.T.);
#6976=ORIENTED_EDGE('',*,*,#5043,.T.);
#6977=ORIENTED_EDGE('',*,*,#5037,.F.);
#6978=ORIENTED_EDGE('',*,*,#5047,.T.);
#6979=ORIENTED_EDGE('',*,*,#5050,.T.);
#6980=ORIENTED_EDGE('',*,*,#5051,.T.);
#6981=ORIENTED_EDGE('',*,*,#5031,.F.);
#6982=ORIENTED_EDGE('',*,*,#5052,.T.);
#6983=ORIENTED_EDGE('',*,*,#5053,.T.);
#6984=ORIENTED_EDGE('',*,*,#5054,.T.);
#6985=ORIENTED_EDGE('',*,*,#5055,.F.);
#6986=ORIENTED_EDGE('',*,*,#5056,.T.);
#6987=ORIENTED_EDGE('',*,*,#5057,.T.);
#6988=ORIENTED_EDGE('',*,*,#5058,.F.);
#6989=ORIENTED_EDGE('',*,*,#5059,.F.);
#6990=ORIENTED_EDGE('',*,*,#5060,.T.);
#6991=ORIENTED_EDGE('',*,*,#5061,.T.);
#6992=ORIENTED_EDGE('',*,*,#5056,.F.);
#6993=ORIENTED_EDGE('',*,*,#5062,.F.);
#6994=ORIENTED_EDGE('',*,*,#5063,.T.);
#6995=ORIENTED_EDGE('',*,*,#5064,.T.);
#6996=ORIENTED_EDGE('',*,*,#5060,.F.);
#6997=ORIENTED_EDGE('',*,*,#5065,.F.);
#6998=ORIENTED_EDGE('',*,*,#5066,.T.);
#6999=ORIENTED_EDGE('',*,*,#5067,.T.);
#7000=ORIENTED_EDGE('',*,*,#5063,.F.);
#7001=ORIENTED_EDGE('',*,*,#5068,.F.);
#7002=ORIENTED_EDGE('',*,*,#5069,.T.);
#7003=ORIENTED_EDGE('',*,*,#5070,.T.);
#7004=ORIENTED_EDGE('',*,*,#5066,.F.);
#7005=ORIENTED_EDGE('',*,*,#5071,.F.);
#7006=ORIENTED_EDGE('',*,*,#5058,.T.);
#7007=ORIENTED_EDGE('',*,*,#5072,.T.);
#7008=ORIENTED_EDGE('',*,*,#5069,.F.);
#7009=ORIENTED_EDGE('',*,*,#5072,.F.);
#7010=ORIENTED_EDGE('',*,*,#5057,.F.);
#7011=ORIENTED_EDGE('',*,*,#5061,.F.);
#7012=ORIENTED_EDGE('',*,*,#5064,.F.);
#7013=ORIENTED_EDGE('',*,*,#5067,.F.);
#7014=ORIENTED_EDGE('',*,*,#5070,.F.);
#7015=ORIENTED_EDGE('',*,*,#5073,.F.);
#7016=ORIENTED_EDGE('',*,*,#5074,.F.);
#7017=ORIENTED_EDGE('',*,*,#5075,.T.);
#7018=ORIENTED_EDGE('',*,*,#5076,.T.);
#7019=ORIENTED_EDGE('',*,*,#5077,.F.);
#7020=ORIENTED_EDGE('',*,*,#5078,.F.);
#7021=ORIENTED_EDGE('',*,*,#5079,.T.);
#7022=ORIENTED_EDGE('',*,*,#5080,.T.);
#7023=ORIENTED_EDGE('',*,*,#5075,.F.);
#7024=ORIENTED_EDGE('',*,*,#5081,.F.);
#7025=ORIENTED_EDGE('',*,*,#5082,.T.);
#7026=ORIENTED_EDGE('',*,*,#5083,.T.);
#7027=ORIENTED_EDGE('',*,*,#5079,.F.);
#7028=ORIENTED_EDGE('',*,*,#5084,.F.);
#7029=ORIENTED_EDGE('',*,*,#5085,.T.);
#7030=ORIENTED_EDGE('',*,*,#5086,.T.);
#7031=ORIENTED_EDGE('',*,*,#5082,.F.);
#7032=ORIENTED_EDGE('',*,*,#5087,.F.);
#7033=ORIENTED_EDGE('',*,*,#5088,.T.);
#7034=ORIENTED_EDGE('',*,*,#5089,.T.);
#7035=ORIENTED_EDGE('',*,*,#5085,.F.);
#7036=ORIENTED_EDGE('',*,*,#5090,.F.);
#7037=ORIENTED_EDGE('',*,*,#5077,.T.);
#7038=ORIENTED_EDGE('',*,*,#5091,.T.);
#7039=ORIENTED_EDGE('',*,*,#5088,.F.);
#7040=ORIENTED_EDGE('',*,*,#5091,.F.);
#7041=ORIENTED_EDGE('',*,*,#5076,.F.);
#7042=ORIENTED_EDGE('',*,*,#5080,.F.);
#7043=ORIENTED_EDGE('',*,*,#5083,.F.);
#7044=ORIENTED_EDGE('',*,*,#5086,.F.);
#7045=ORIENTED_EDGE('',*,*,#5089,.F.);
#7046=ORIENTED_EDGE('',*,*,#5092,.F.);
#7047=ORIENTED_EDGE('',*,*,#5093,.F.);
#7048=ORIENTED_EDGE('',*,*,#5094,.T.);
#7049=ORIENTED_EDGE('',*,*,#5052,.F.);
#7050=ORIENTED_EDGE('',*,*,#5094,.F.);
#7051=ORIENTED_EDGE('',*,*,#5095,.F.);
#7052=ORIENTED_EDGE('',*,*,#5096,.T.);
#7053=ORIENTED_EDGE('',*,*,#5097,.F.);
#7054=ORIENTED_EDGE('',*,*,#5096,.F.);
#7055=ORIENTED_EDGE('',*,*,#5098,.F.);
#7056=ORIENTED_EDGE('',*,*,#5099,.T.);
#7057=ORIENTED_EDGE('',*,*,#5100,.F.);
#7058=ORIENTED_EDGE('',*,*,#5099,.F.);
#7059=ORIENTED_EDGE('',*,*,#5101,.F.);
#7060=ORIENTED_EDGE('',*,*,#5102,.T.);
#7061=ORIENTED_EDGE('',*,*,#5053,.F.);
#7062=ORIENTED_EDGE('',*,*,#5102,.F.);
#7063=ORIENTED_EDGE('',*,*,#5092,.T.);
#7064=ORIENTED_EDGE('',*,*,#5103,.T.);
#7065=ORIENTED_EDGE('',*,*,#5104,.F.);
#7066=ORIENTED_EDGE('',*,*,#5103,.F.);
#7067=ORIENTED_EDGE('',*,*,#5073,.T.);
#7068=ORIENTED_EDGE('',*,*,#5105,.T.);
#7069=ORIENTED_EDGE('',*,*,#5106,.F.);
#7070=ORIENTED_EDGE('',*,*,#5105,.F.);
#7071=ORIENTED_EDGE('',*,*,#5107,.F.);
#7072=ORIENTED_EDGE('',*,*,#5108,.F.);
#7073=ORIENTED_EDGE('',*,*,#5109,.F.);
#7074=ORIENTED_EDGE('',*,*,#5110,.T.);
#7075=ORIENTED_EDGE('',*,*,#5111,.F.);
#7076=ORIENTED_EDGE('',*,*,#5112,.T.);
#7077=ORIENTED_EDGE('',*,*,#5113,.F.);
#7078=ORIENTED_EDGE('',*,*,#5114,.F.);
#7079=ORIENTED_EDGE('',*,*,#5115,.F.);
#7080=ORIENTED_EDGE('',*,*,#5116,.T.);
#7081=ORIENTED_EDGE('',*,*,#5117,.F.);
#7082=ORIENTED_EDGE('',*,*,#5118,.F.);
#7083=ORIENTED_EDGE('',*,*,#5119,.F.);
#7084=ORIENTED_EDGE('',*,*,#5120,.T.);
#7085=ORIENTED_EDGE('',*,*,#5121,.F.);
#7086=ORIENTED_EDGE('',*,*,#5122,.F.);
#7087=ORIENTED_EDGE('',*,*,#5123,.F.);
#7088=ORIENTED_EDGE('',*,*,#5124,.T.);
#7089=ORIENTED_EDGE('',*,*,#5125,.F.);
#7090=ORIENTED_EDGE('',*,*,#5126,.F.);
#7091=ORIENTED_EDGE('',*,*,#5127,.F.);
#7092=ORIENTED_EDGE('',*,*,#5128,.F.);
#7093=ORIENTED_EDGE('',*,*,#5129,.F.);
#7094=ORIENTED_EDGE('',*,*,#5130,.T.);
#7095=ORIENTED_EDGE('',*,*,#5131,.F.);
#7096=ORIENTED_EDGE('',*,*,#5132,.F.);
#7097=ORIENTED_EDGE('',*,*,#5133,.F.);
#7098=ORIENTED_EDGE('',*,*,#5134,.T.);
#7099=ORIENTED_EDGE('',*,*,#5135,.F.);
#7100=ORIENTED_EDGE('',*,*,#5104,.T.);
#7101=ORIENTED_EDGE('',*,*,#5136,.F.);
#7102=ORIENTED_EDGE('',*,*,#5106,.T.);
#7103=ORIENTED_EDGE('',*,*,#5137,.F.);
#7104=ORIENTED_EDGE('',*,*,#5110,.F.);
#7105=ORIENTED_EDGE('',*,*,#5138,.F.);
#7106=ORIENTED_EDGE('',*,*,#5124,.F.);
#7107=ORIENTED_EDGE('',*,*,#5139,.F.);
#7108=ORIENTED_EDGE('',*,*,#5130,.F.);
#7109=ORIENTED_EDGE('',*,*,#5140,.F.);
#7110=ORIENTED_EDGE('',*,*,#5112,.F.);
#7111=ORIENTED_EDGE('',*,*,#5141,.F.);
#7112=ORIENTED_EDGE('',*,*,#5134,.F.);
#7113=ORIENTED_EDGE('',*,*,#5142,.F.);
#7114=ORIENTED_EDGE('',*,*,#5116,.F.);
#7115=ORIENTED_EDGE('',*,*,#5143,.F.);
#7116=ORIENTED_EDGE('',*,*,#5144,.F.);
#7117=ORIENTED_EDGE('',*,*,#5145,.F.);
#7118=ORIENTED_EDGE('',*,*,#5120,.F.);
#7119=ORIENTED_EDGE('',*,*,#5146,.F.);
#7120=ORIENTED_EDGE('',*,*,#5147,.F.);
#7121=ORIENTED_EDGE('',*,*,#5148,.F.);
#7122=ORIENTED_EDGE('',*,*,#5144,.T.);
#7123=ORIENTED_EDGE('',*,*,#5149,.T.);
#7124=ORIENTED_EDGE('',*,*,#5150,.F.);
#7125=ORIENTED_EDGE('',*,*,#5151,.F.);
#7126=ORIENTED_EDGE('',*,*,#5050,.F.);
#7127=ORIENTED_EDGE('',*,*,#5046,.F.);
#7128=ORIENTED_EDGE('',*,*,#5152,.F.);
#7129=ORIENTED_EDGE('',*,*,#5121,.T.);
#7130=ORIENTED_EDGE('',*,*,#5145,.T.);
#7131=ORIENTED_EDGE('',*,*,#5148,.T.);
#7132=ORIENTED_EDGE('',*,*,#5153,.T.);
#7133=ORIENTED_EDGE('',*,*,#5154,.F.);
#7134=ORIENTED_EDGE('',*,*,#5044,.F.);
#7135=ORIENTED_EDGE('',*,*,#5049,.F.);
#7136=ORIENTED_EDGE('',*,*,#5155,.F.);
#7137=ORIENTED_EDGE('',*,*,#5156,.F.);
#7138=ORIENTED_EDGE('',*,*,#5157,.T.);
#7139=ORIENTED_EDGE('',*,*,#5117,.T.);
#7140=ORIENTED_EDGE('',*,*,#5142,.T.);
#7141=ORIENTED_EDGE('',*,*,#5133,.T.);
#7142=ORIENTED_EDGE('',*,*,#5158,.T.);
#7143=ORIENTED_EDGE('',*,*,#5159,.F.);
#7144=ORIENTED_EDGE('',*,*,#5160,.F.);
#7145=ORIENTED_EDGE('',*,*,#5161,.F.);
#7146=ORIENTED_EDGE('',*,*,#5162,.F.);
#7147=ORIENTED_EDGE('',*,*,#5163,.F.);
#7148=ORIENTED_EDGE('',*,*,#5164,.T.);
#7149=ORIENTED_EDGE('',*,*,#5113,.T.);
#7150=ORIENTED_EDGE('',*,*,#5140,.T.);
#7151=ORIENTED_EDGE('',*,*,#5129,.T.);
#7152=ORIENTED_EDGE('',*,*,#5165,.T.);
#7153=ORIENTED_EDGE('',*,*,#5166,.F.);
#7154=ORIENTED_EDGE('',*,*,#5039,.F.);
#7155=ORIENTED_EDGE('',*,*,#5167,.F.);
#7156=ORIENTED_EDGE('',*,*,#5168,.F.);
#7157=ORIENTED_EDGE('',*,*,#5169,.F.);
#7158=ORIENTED_EDGE('',*,*,#5170,.T.);
#7159=ORIENTED_EDGE('',*,*,#5107,.T.);
#7160=ORIENTED_EDGE('',*,*,#5137,.T.);
#7161=ORIENTED_EDGE('',*,*,#5123,.T.);
#7162=ORIENTED_EDGE('',*,*,#5171,.F.);
#7163=ORIENTED_EDGE('',*,*,#5172,.T.);
#7164=ORIENTED_EDGE('',*,*,#5173,.T.);
#7165=ORIENTED_EDGE('',*,*,#5174,.T.);
#7166=ORIENTED_EDGE('',*,*,#5175,.F.);
#7167=ORIENTED_EDGE('',*,*,#5122,.T.);
#7168=ORIENTED_EDGE('',*,*,#5157,.F.);
#7169=ORIENTED_EDGE('',*,*,#5176,.T.);
#7170=ORIENTED_EDGE('',*,*,#5149,.F.);
#7171=ORIENTED_EDGE('',*,*,#5177,.T.);
#7172=ORIENTED_EDGE('',*,*,#5153,.F.);
#7173=ORIENTED_EDGE('',*,*,#5147,.T.);
#7174=ORIENTED_EDGE('',*,*,#5178,.F.);
#7175=ORIENTED_EDGE('',*,*,#5179,.T.);
#7176=ORIENTED_EDGE('',*,*,#5158,.F.);
#7177=ORIENTED_EDGE('',*,*,#5132,.T.);
#7178=ORIENTED_EDGE('',*,*,#5180,.F.);
#7179=ORIENTED_EDGE('',*,*,#5181,.T.);
#7180=ORIENTED_EDGE('',*,*,#5165,.F.);
#7181=ORIENTED_EDGE('',*,*,#5128,.T.);
#7182=ORIENTED_EDGE('',*,*,#5182,.F.);
#7183=ORIENTED_EDGE('',*,*,#5183,.T.);
#7184=ORIENTED_EDGE('',*,*,#5184,.T.);
#7185=ORIENTED_EDGE('',*,*,#5171,.T.);
#7186=ORIENTED_EDGE('',*,*,#5126,.T.);
#7187=ORIENTED_EDGE('',*,*,#5185,.T.);
#7188=ORIENTED_EDGE('',*,*,#5186,.F.);
#7189=ORIENTED_EDGE('',*,*,#5187,.T.);
#7190=ORIENTED_EDGE('',*,*,#5188,.F.);
#7191=ORIENTED_EDGE('',*,*,#5189,.T.);
#7192=ORIENTED_EDGE('',*,*,#5190,.F.);
#7193=ORIENTED_EDGE('',*,*,#5191,.T.);
#7194=ORIENTED_EDGE('',*,*,#5192,.F.);
#7195=ORIENTED_EDGE('',*,*,#5193,.T.);
#7196=ORIENTED_EDGE('',*,*,#5108,.T.);
#7197=ORIENTED_EDGE('',*,*,#5175,.T.);
#7198=ORIENTED_EDGE('',*,*,#5194,.T.);
#7199=ORIENTED_EDGE('',*,*,#5195,.T.);
#7200=ORIENTED_EDGE('',*,*,#5196,.F.);
#7201=ORIENTED_EDGE('',*,*,#5114,.T.);
#7202=ORIENTED_EDGE('',*,*,#5170,.F.);
#7203=ORIENTED_EDGE('',*,*,#5197,.T.);
#7204=ORIENTED_EDGE('',*,*,#5198,.F.);
#7205=ORIENTED_EDGE('',*,*,#5118,.T.);
#7206=ORIENTED_EDGE('',*,*,#5164,.F.);
#7207=ORIENTED_EDGE('',*,*,#5199,.T.);
#7208=ORIENTED_EDGE('',*,*,#5200,.F.);
#7209=ORIENTED_EDGE('',*,*,#5201,.T.);
#7210=ORIENTED_EDGE('',*,*,#5202,.T.);
#7211=ORIENTED_EDGE('',*,*,#5203,.T.);
#7212=ORIENTED_EDGE('',*,*,#5204,.T.);
#7213=ORIENTED_EDGE('',*,*,#5205,.T.);
#7214=ORIENTED_EDGE('',*,*,#5206,.F.);
#7215=ORIENTED_EDGE('',*,*,#5054,.F.);
#7216=ORIENTED_EDGE('',*,*,#5207,.T.);
#7217=ORIENTED_EDGE('',*,*,#5136,.T.);
#7218=ORIENTED_EDGE('',*,*,#5207,.F.);
#7219=ORIENTED_EDGE('',*,*,#5208,.F.);
#7220=ORIENTED_EDGE('',*,*,#5209,.T.);
#7221=ORIENTED_EDGE('',*,*,#5135,.T.);
#7222=ORIENTED_EDGE('',*,*,#5209,.F.);
#7223=ORIENTED_EDGE('',*,*,#5210,.F.);
#7224=ORIENTED_EDGE('',*,*,#5206,.T.);
#7225=ORIENTED_EDGE('',*,*,#5211,.F.);
#7226=ORIENTED_EDGE('',*,*,#5212,.F.);
#7227=ORIENTED_EDGE('',*,*,#5213,.F.);
#7228=ORIENTED_EDGE('',*,*,#5214,.F.);
#7229=ORIENTED_EDGE('',*,*,#5150,.T.);
#7230=ORIENTED_EDGE('',*,*,#5176,.F.);
#7231=ORIENTED_EDGE('',*,*,#5156,.T.);
#7232=ORIENTED_EDGE('',*,*,#5215,.T.);
#7233=ORIENTED_EDGE('',*,*,#5210,.T.);
#7234=ORIENTED_EDGE('',*,*,#5216,.T.);
#7235=ORIENTED_EDGE('',*,*,#5217,.T.);
#7236=ORIENTED_EDGE('',*,*,#5201,.F.);
#7237=ORIENTED_EDGE('',*,*,#5030,.T.);
#7238=ORIENTED_EDGE('',*,*,#5051,.F.);
#7239=ORIENTED_EDGE('',*,*,#5151,.T.);
#7240=ORIENTED_EDGE('',*,*,#5215,.F.);
#7241=ORIENTED_EDGE('',*,*,#5155,.T.);
#7242=ORIENTED_EDGE('',*,*,#5048,.F.);
#7243=ORIENTED_EDGE('',*,*,#5214,.T.);
#7244=ORIENTED_EDGE('',*,*,#5218,.F.);
#7245=ORIENTED_EDGE('',*,*,#5219,.F.);
#7246=ORIENTED_EDGE('',*,*,#5216,.F.);
#7247=ORIENTED_EDGE('',*,*,#5213,.T.);
#7248=ORIENTED_EDGE('',*,*,#5220,.T.);
#7249=ORIENTED_EDGE('',*,*,#5221,.T.);
#7250=ORIENTED_EDGE('',*,*,#5218,.T.);
#7251=ORIENTED_EDGE('',*,*,#5152,.T.);
#7252=ORIENTED_EDGE('',*,*,#5045,.T.);
#7253=ORIENTED_EDGE('',*,*,#5154,.T.);
#7254=ORIENTED_EDGE('',*,*,#5177,.F.);
#7255=ORIENTED_EDGE('',*,*,#5211,.T.);
#7256=ORIENTED_EDGE('',*,*,#5205,.F.);
#7257=ORIENTED_EDGE('',*,*,#5222,.T.);
#7258=ORIENTED_EDGE('',*,*,#5223,.T.);
#7259=ORIENTED_EDGE('',*,*,#5119,.T.);
#7260=ORIENTED_EDGE('',*,*,#5200,.T.);
#7261=ORIENTED_EDGE('',*,*,#5224,.F.);
#7262=ORIENTED_EDGE('',*,*,#5225,.F.);
#7263=ORIENTED_EDGE('',*,*,#5226,.F.);
#7264=ORIENTED_EDGE('',*,*,#5227,.F.);
#7265=ORIENTED_EDGE('',*,*,#5228,.F.);
#7266=ORIENTED_EDGE('',*,*,#5178,.T.);
#7267=ORIENTED_EDGE('',*,*,#5146,.T.);
#7268=ORIENTED_EDGE('',*,*,#5143,.T.);
#7269=ORIENTED_EDGE('',*,*,#5224,.T.);
#7270=ORIENTED_EDGE('',*,*,#5199,.F.);
#7271=ORIENTED_EDGE('',*,*,#5163,.T.);
#7272=ORIENTED_EDGE('',*,*,#5229,.T.);
#7273=ORIENTED_EDGE('',*,*,#5225,.T.);
#7274=ORIENTED_EDGE('',*,*,#5229,.F.);
#7275=ORIENTED_EDGE('',*,*,#5162,.T.);
#7276=ORIENTED_EDGE('',*,*,#5230,.F.);
#7277=ORIENTED_EDGE('',*,*,#5226,.T.);
#7278=ORIENTED_EDGE('',*,*,#5230,.T.);
#7279=ORIENTED_EDGE('',*,*,#5161,.T.);
#7280=ORIENTED_EDGE('',*,*,#5231,.T.);
#7281=ORIENTED_EDGE('',*,*,#5227,.T.);
#7282=ORIENTED_EDGE('',*,*,#5231,.F.);
#7283=ORIENTED_EDGE('',*,*,#5160,.T.);
#7284=ORIENTED_EDGE('',*,*,#5232,.F.);
#7285=ORIENTED_EDGE('',*,*,#5228,.T.);
#7286=ORIENTED_EDGE('',*,*,#5232,.T.);
#7287=ORIENTED_EDGE('',*,*,#5159,.T.);
#7288=ORIENTED_EDGE('',*,*,#5179,.F.);
#7289=ORIENTED_EDGE('',*,*,#5115,.T.);
#7290=ORIENTED_EDGE('',*,*,#5198,.T.);
#7291=ORIENTED_EDGE('',*,*,#5233,.F.);
#7292=ORIENTED_EDGE('',*,*,#5234,.F.);
#7293=ORIENTED_EDGE('',*,*,#5235,.F.);
#7294=ORIENTED_EDGE('',*,*,#5041,.F.);
#7295=ORIENTED_EDGE('',*,*,#5236,.F.);
#7296=ORIENTED_EDGE('',*,*,#5180,.T.);
#7297=ORIENTED_EDGE('',*,*,#5131,.T.);
#7298=ORIENTED_EDGE('',*,*,#5141,.T.);
#7299=ORIENTED_EDGE('',*,*,#5233,.T.);
#7300=ORIENTED_EDGE('',*,*,#5197,.F.);
#7301=ORIENTED_EDGE('',*,*,#5169,.T.);
#7302=ORIENTED_EDGE('',*,*,#5237,.T.);
#7303=ORIENTED_EDGE('',*,*,#5034,.T.);
#7304=ORIENTED_EDGE('',*,*,#5238,.F.);
#7305=ORIENTED_EDGE('',*,*,#5234,.T.);
#7306=ORIENTED_EDGE('',*,*,#5237,.F.);
#7307=ORIENTED_EDGE('',*,*,#5168,.T.);
#7308=ORIENTED_EDGE('',*,*,#5239,.F.);
#7309=ORIENTED_EDGE('',*,*,#5042,.T.);
#7310=ORIENTED_EDGE('',*,*,#5235,.T.);
#7311=ORIENTED_EDGE('',*,*,#5238,.T.);
#7312=ORIENTED_EDGE('',*,*,#5035,.F.);
#7313=ORIENTED_EDGE('',*,*,#5239,.T.);
#7314=ORIENTED_EDGE('',*,*,#5167,.T.);
#7315=ORIENTED_EDGE('',*,*,#5038,.T.);
#7316=ORIENTED_EDGE('',*,*,#5033,.F.);
#7317=ORIENTED_EDGE('',*,*,#5100,.T.);
#7318=ORIENTED_EDGE('',*,*,#5097,.T.);
#7319=ORIENTED_EDGE('',*,*,#5208,.T.);
#7320=ORIENTED_EDGE('',*,*,#5236,.T.);
#7321=ORIENTED_EDGE('',*,*,#5040,.T.);
#7322=ORIENTED_EDGE('',*,*,#5166,.T.);
#7323=ORIENTED_EDGE('',*,*,#5181,.F.);
#7324=ORIENTED_EDGE('',*,*,#5111,.T.);
#7325=ORIENTED_EDGE('',*,*,#5196,.T.);
#7326=ORIENTED_EDGE('',*,*,#5240,.F.);
#7327=ORIENTED_EDGE('',*,*,#5241,.F.);
#7328=ORIENTED_EDGE('',*,*,#5242,.F.);
#7329=ORIENTED_EDGE('',*,*,#5243,.F.);
#7330=ORIENTED_EDGE('',*,*,#5244,.F.);
#7331=ORIENTED_EDGE('',*,*,#5182,.T.);
#7332=ORIENTED_EDGE('',*,*,#5127,.T.);
#7333=ORIENTED_EDGE('',*,*,#5139,.T.);
#7334=ORIENTED_EDGE('',*,*,#5240,.T.);
#7335=ORIENTED_EDGE('',*,*,#5195,.F.);
#7336=ORIENTED_EDGE('',*,*,#5245,.T.);
#7337=ORIENTED_EDGE('',*,*,#5246,.T.);
#7338=ORIENTED_EDGE('',*,*,#5241,.T.);
#7339=ORIENTED_EDGE('',*,*,#5246,.F.);
#7340=ORIENTED_EDGE('',*,*,#5247,.F.);
#7341=ORIENTED_EDGE('',*,*,#5248,.F.);
#7342=ORIENTED_EDGE('',*,*,#5242,.T.);
#7343=ORIENTED_EDGE('',*,*,#5248,.T.);
#7344=ORIENTED_EDGE('',*,*,#5249,.T.);
#7345=ORIENTED_EDGE('',*,*,#5250,.T.);
#7346=ORIENTED_EDGE('',*,*,#5244,.T.);
#7347=ORIENTED_EDGE('',*,*,#5251,.T.);
#7348=ORIENTED_EDGE('',*,*,#5252,.T.);
#7349=ORIENTED_EDGE('',*,*,#5183,.F.);
#7350=ORIENTED_EDGE('',*,*,#5243,.T.);
#7351=ORIENTED_EDGE('',*,*,#5250,.F.);
#7352=ORIENTED_EDGE('',*,*,#5253,.F.);
#7353=ORIENTED_EDGE('',*,*,#5251,.F.);
#7354=ORIENTED_EDGE('',*,*,#5254,.T.);
#7355=ORIENTED_EDGE('',*,*,#5255,.T.);
#7356=ORIENTED_EDGE('',*,*,#5253,.T.);
#7357=ORIENTED_EDGE('',*,*,#5256,.T.);
#7358=ORIENTED_EDGE('',*,*,#5257,.T.);
#7359=ORIENTED_EDGE('',*,*,#5258,.T.);
#7360=ORIENTED_EDGE('',*,*,#5247,.T.);
#7361=ORIENTED_EDGE('',*,*,#5259,.T.);
#7362=ORIENTED_EDGE('',*,*,#5260,.T.);
#7363=ORIENTED_EDGE('',*,*,#5254,.F.);
#7364=ORIENTED_EDGE('',*,*,#5249,.F.);
#7365=ORIENTED_EDGE('',*,*,#5260,.F.);
#7366=ORIENTED_EDGE('',*,*,#5173,.F.);
#7367=ORIENTED_EDGE('',*,*,#5194,.F.);
#7368=ORIENTED_EDGE('',*,*,#5174,.F.);
#7369=ORIENTED_EDGE('',*,*,#5259,.F.);
#7370=ORIENTED_EDGE('',*,*,#5245,.F.);
#7371=ORIENTED_EDGE('',*,*,#5261,.T.);
#7372=ORIENTED_EDGE('',*,*,#5219,.T.);
#7373=ORIENTED_EDGE('',*,*,#5262,.T.);
#7374=ORIENTED_EDGE('',*,*,#5262,.F.);
#7375=ORIENTED_EDGE('',*,*,#5221,.F.);
#7376=ORIENTED_EDGE('',*,*,#5258,.F.);
#7377=ORIENTED_EDGE('',*,*,#5263,.F.);
#7378=ORIENTED_EDGE('',*,*,#5202,.F.);
#7379=ORIENTED_EDGE('',*,*,#5217,.F.);
#7380=ORIENTED_EDGE('',*,*,#5261,.F.);
#7381=ORIENTED_EDGE('',*,*,#5264,.F.);
#7382=ORIENTED_EDGE('',*,*,#5204,.F.);
#7383=ORIENTED_EDGE('',*,*,#5265,.F.);
#7384=ORIENTED_EDGE('',*,*,#5257,.F.);
#7385=ORIENTED_EDGE('',*,*,#5222,.F.);
#7386=ORIENTED_EDGE('',*,*,#5212,.T.);
#7387=ORIENTED_EDGE('',*,*,#5223,.F.);
#7388=ORIENTED_EDGE('',*,*,#5256,.F.);
#7389=ORIENTED_EDGE('',*,*,#5220,.F.);
#7390=ORIENTED_EDGE('',*,*,#5184,.F.);
#7391=ORIENTED_EDGE('',*,*,#5252,.F.);
#7392=ORIENTED_EDGE('',*,*,#5255,.F.);
#7393=ORIENTED_EDGE('',*,*,#5172,.F.);
#7394=ORIENTED_EDGE('',*,*,#5264,.T.);
#7395=ORIENTED_EDGE('',*,*,#5263,.T.);
#7396=ORIENTED_EDGE('',*,*,#5265,.T.);
#7397=ORIENTED_EDGE('',*,*,#5203,.F.);
#7398=ORIENTED_EDGE('',*,*,#5266,.F.);
#7399=ORIENTED_EDGE('',*,*,#5267,.F.);
#7400=ORIENTED_EDGE('',*,*,#5268,.F.);
#7401=ORIENTED_EDGE('',*,*,#5269,.F.);
#7402=ORIENTED_EDGE('',*,*,#5270,.F.);
#7403=ORIENTED_EDGE('',*,*,#5271,.F.);
#7404=ORIENTED_EDGE('',*,*,#5272,.F.);
#7405=ORIENTED_EDGE('',*,*,#5273,.F.);
#7406=ORIENTED_EDGE('',*,*,#5274,.F.);
#7407=ORIENTED_EDGE('',*,*,#5266,.T.);
#7408=ORIENTED_EDGE('',*,*,#5275,.T.);
#7409=ORIENTED_EDGE('',*,*,#5273,.T.);
#7410=ORIENTED_EDGE('',*,*,#5276,.T.);
#7411=ORIENTED_EDGE('',*,*,#5192,.T.);
#7412=ORIENTED_EDGE('',*,*,#5277,.T.);
#7413=ORIENTED_EDGE('',*,*,#5274,.T.);
#7414=ORIENTED_EDGE('',*,*,#5278,.T.);
#7415=ORIENTED_EDGE('',*,*,#5279,.F.);
#7416=ORIENTED_EDGE('',*,*,#5280,.F.);
#7417=ORIENTED_EDGE('',*,*,#5281,.F.);
#7418=ORIENTED_EDGE('',*,*,#5280,.T.);
#7419=ORIENTED_EDGE('',*,*,#5282,.T.);
#7420=ORIENTED_EDGE('',*,*,#5270,.T.);
#7421=ORIENTED_EDGE('',*,*,#5283,.T.);
#7422=ORIENTED_EDGE('',*,*,#5272,.T.);
#7423=ORIENTED_EDGE('',*,*,#5284,.T.);
#7424=ORIENTED_EDGE('',*,*,#5281,.T.);
#7425=ORIENTED_EDGE('',*,*,#5285,.T.);
#7426=ORIENTED_EDGE('',*,*,#5190,.T.);
#7427=ORIENTED_EDGE('',*,*,#5286,.T.);
#7428=ORIENTED_EDGE('',*,*,#5279,.T.);
#7429=ORIENTED_EDGE('',*,*,#5287,.T.);
#7430=ORIENTED_EDGE('',*,*,#5188,.T.);
#7431=ORIENTED_EDGE('',*,*,#5288,.T.);
#7432=ORIENTED_EDGE('',*,*,#5271,.T.);
#7433=ORIENTED_EDGE('',*,*,#5289,.T.);
#7434=ORIENTED_EDGE('',*,*,#5269,.T.);
#7435=ORIENTED_EDGE('',*,*,#5290,.T.);
#7436=ORIENTED_EDGE('',*,*,#5267,.T.);
#7437=ORIENTED_EDGE('',*,*,#5291,.T.);
#7438=ORIENTED_EDGE('',*,*,#5186,.T.);
#7439=ORIENTED_EDGE('',*,*,#5292,.T.);
#7440=ORIENTED_EDGE('',*,*,#5268,.T.);
#7441=ORIENTED_EDGE('',*,*,#5293,.T.);
#7442=ORIENTED_EDGE('',*,*,#5287,.F.);
#7443=ORIENTED_EDGE('',*,*,#5284,.F.);
#7444=ORIENTED_EDGE('',*,*,#5277,.F.);
#7445=ORIENTED_EDGE('',*,*,#5191,.F.);
#7446=ORIENTED_EDGE('',*,*,#5109,.T.);
#7447=ORIENTED_EDGE('',*,*,#5193,.F.);
#7448=ORIENTED_EDGE('',*,*,#5278,.F.);
#7449=ORIENTED_EDGE('',*,*,#5275,.F.);
#7450=ORIENTED_EDGE('',*,*,#5292,.F.);
#7451=ORIENTED_EDGE('',*,*,#5185,.F.);
#7452=ORIENTED_EDGE('',*,*,#5125,.T.);
#7453=ORIENTED_EDGE('',*,*,#5138,.T.);
#7454=ORIENTED_EDGE('',*,*,#5283,.F.);
#7455=ORIENTED_EDGE('',*,*,#5291,.F.);
#7456=ORIENTED_EDGE('',*,*,#5276,.F.);
#7457=ORIENTED_EDGE('',*,*,#5285,.F.);
#7458=ORIENTED_EDGE('',*,*,#5055,.T.);
#7459=ORIENTED_EDGE('',*,*,#5071,.T.);
#7460=ORIENTED_EDGE('',*,*,#5068,.T.);
#7461=ORIENTED_EDGE('',*,*,#5065,.T.);
#7462=ORIENTED_EDGE('',*,*,#5062,.T.);
#7463=ORIENTED_EDGE('',*,*,#5059,.T.);
#7464=ORIENTED_EDGE('',*,*,#5074,.T.);
#7465=ORIENTED_EDGE('',*,*,#5090,.T.);
#7466=ORIENTED_EDGE('',*,*,#5087,.T.);
#7467=ORIENTED_EDGE('',*,*,#5084,.T.);
#7468=ORIENTED_EDGE('',*,*,#5081,.T.);
#7469=ORIENTED_EDGE('',*,*,#5078,.T.);
#7470=ORIENTED_EDGE('',*,*,#5101,.T.);
#7471=ORIENTED_EDGE('',*,*,#5098,.T.);
#7472=ORIENTED_EDGE('',*,*,#5095,.T.);
#7473=ORIENTED_EDGE('',*,*,#5093,.T.);
#7474=ORIENTED_EDGE('',*,*,#5288,.F.);
#7475=ORIENTED_EDGE('',*,*,#5187,.F.);
#7476=ORIENTED_EDGE('',*,*,#5293,.F.);
#7477=ORIENTED_EDGE('',*,*,#5290,.F.);
#7478=ORIENTED_EDGE('',*,*,#5286,.F.);
#7479=ORIENTED_EDGE('',*,*,#5189,.F.);
#7480=ORIENTED_EDGE('',*,*,#5289,.F.);
#7481=ORIENTED_EDGE('',*,*,#5282,.F.);
#8215=CYLINDRICAL_SURFACE('',#9199,0.25);
#8216=CYLINDRICAL_SURFACE('',#9201,0.25);
#8217=CYLINDRICAL_SURFACE('',#9203,0.25);
#8218=CYLINDRICAL_SURFACE('',#9205,0.25);
#8219=CYLINDRICAL_SURFACE('',#9227,0.15);
#8220=CYLINDRICAL_SURFACE('',#9229,0.15);
#8221=CYLINDRICAL_SURFACE('',#9232,0.15);
#8222=CYLINDRICAL_SURFACE('',#9235,0.15);
#8223=CYLINDRICAL_SURFACE('',#9237,0.17);
#8224=CYLINDRICAL_SURFACE('',#9239,0.17);
#8225=CYLINDRICAL_SURFACE('',#9263,0.4);
#8226=CYLINDRICAL_SURFACE('',#9264,0.4);
#8227=CYLINDRICAL_SURFACE('',#9287,0.1);
#8228=CYLINDRICAL_SURFACE('',#9291,0.1);
#8229=CYLINDRICAL_SURFACE('',#9305,0.3);
#8230=CYLINDRICAL_SURFACE('',#9310,0.3);
#8562=ADVANCED_FACE('',(#1145),#8215,.F.);
#8563=ADVANCED_FACE('',(#1146),#8216,.F.);
#8564=ADVANCED_FACE('',(#1147),#8217,.F.);
#8565=ADVANCED_FACE('',(#1148),#8218,.F.);
#8566=ADVANCED_FACE('',(#1149),#124,.T.);
#8567=ADVANCED_FACE('',(#1150),#125,.T.);
#8568=ADVANCED_FACE('',(#1151,#616,#617,#618),#824,.F.);
#8569=ADVANCED_FACE('',(#1152),#825,.F.);
#8570=ADVANCED_FACE('',(#1153),#826,.F.);
#8571=ADVANCED_FACE('',(#1154),#827,.F.);
#8572=ADVANCED_FACE('',(#1155),#828,.F.);
#8573=ADVANCED_FACE('',(#1156),#829,.F.);
#8574=ADVANCED_FACE('',(#1157),#830,.F.);
#8575=ADVANCED_FACE('',(#1158,#619),#831,.F.);
#8576=ADVANCED_FACE('',(#1159),#832,.F.);
#8577=ADVANCED_FACE('',(#1160),#833,.F.);
#8578=ADVANCED_FACE('',(#1161),#834,.F.);
#8579=ADVANCED_FACE('',(#1162),#835,.F.);
#8580=ADVANCED_FACE('',(#1163),#836,.F.);
#8581=ADVANCED_FACE('',(#1164),#837,.F.);
#8582=ADVANCED_FACE('',(#1165,#620),#838,.F.);
#8583=ADVANCED_FACE('',(#1166),#8219,.F.);
#8584=ADVANCED_FACE('',(#1167),#8220,.F.);
#8585=ADVANCED_FACE('',(#1168),#8221,.F.);
#8586=ADVANCED_FACE('',(#1169),#8222,.F.);
#8587=ADVANCED_FACE('',(#1170),#8223,.F.);
#8588=ADVANCED_FACE('',(#1171),#8224,.F.);
#8589=ADVANCED_FACE('',(#1172),#839,.F.);
#8590=ADVANCED_FACE('',(#1173),#840,.F.);
#8591=ADVANCED_FACE('',(#1174),#841,.F.);
#8592=ADVANCED_FACE('',(#1175),#842,.F.);
#8593=ADVANCED_FACE('',(#1176),#843,.F.);
#8594=ADVANCED_FACE('',(#1177),#844,.F.);
#8595=ADVANCED_FACE('',(#1178),#845,.F.);
#8596=ADVANCED_FACE('',(#1179,#621),#846,.F.);
#8597=ADVANCED_FACE('',(#1180,#622),#847,.F.);
#8598=ADVANCED_FACE('',(#1181),#848,.F.);
#8599=ADVANCED_FACE('',(#1182),#849,.F.);
#8600=ADVANCED_FACE('',(#1183),#850,.F.);
#8601=ADVANCED_FACE('',(#1184),#851,.F.);
#8602=ADVANCED_FACE('',(#1185),#852,.F.);
#8603=ADVANCED_FACE('',(#1186),#853,.T.);
#8604=ADVANCED_FACE('',(#1187),#854,.T.);
#8605=ADVANCED_FACE('',(#1188),#855,.T.);
#8606=ADVANCED_FACE('',(#1189),#856,.T.);
#8607=ADVANCED_FACE('',(#1190),#857,.T.);
#8608=ADVANCED_FACE('',(#1191,#623),#858,.F.);
#8609=ADVANCED_FACE('',(#1192),#8225,.T.);
#8610=ADVANCED_FACE('',(#1193),#8226,.T.);
#8611=ADVANCED_FACE('',(#1194),#859,.T.);
#8612=ADVANCED_FACE('',(#1195),#126,.T.);
#8613=ADVANCED_FACE('',(#1196),#127,.T.);
#8614=ADVANCED_FACE('',(#1197),#128,.T.);
#8615=ADVANCED_FACE('',(#1198),#129,.T.);
#8616=ADVANCED_FACE('',(#1199),#860,.F.);
#8617=ADVANCED_FACE('',(#1200),#130,.T.);
#8618=ADVANCED_FACE('',(#1201),#131,.T.);
#8619=ADVANCED_FACE('',(#1202),#861,.T.);
#8620=ADVANCED_FACE('',(#1203),#132,.T.);
#8621=ADVANCED_FACE('',(#1204),#133,.T.);
#8622=ADVANCED_FACE('',(#1205),#862,.F.);
#8623=ADVANCED_FACE('',(#1206),#134,.T.);
#8624=ADVANCED_FACE('',(#1207),#135,.T.);
#8625=ADVANCED_FACE('',(#1208),#863,.T.);
#8626=ADVANCED_FACE('',(#1209),#136,.T.);
#8627=ADVANCED_FACE('',(#1210),#137,.T.);
#8628=ADVANCED_FACE('',(#1211,#624,#625,#626),#864,.F.);
#8629=ADVANCED_FACE('',(#1212),#138,.T.);
#8630=ADVANCED_FACE('',(#1213),#865,.T.);
#8631=ADVANCED_FACE('',(#1214),#139,.T.);
#8632=ADVANCED_FACE('',(#1215),#140,.T.);
#8633=ADVANCED_FACE('',(#1216),#866,.F.);
#8634=ADVANCED_FACE('',(#1217),#141,.T.);
#8635=ADVANCED_FACE('',(#1218),#142,.T.);
#8636=ADVANCED_FACE('',(#1219),#84,.F.);
#8637=ADVANCED_FACE('',(#1220),#85,.F.);
#8638=ADVANCED_FACE('',(#1221),#86,.F.);
#8639=ADVANCED_FACE('',(#1222),#8227,.F.);
#8640=ADVANCED_FACE('',(#1223),#143,.T.);
#8641=ADVANCED_FACE('',(#1224),#87,.F.);
#8642=ADVANCED_FACE('',(#1225),#8228,.F.);
#8643=ADVANCED_FACE('',(#1226),#144,.T.);
#8644=ADVANCED_FACE('',(#1227),#145,.T.);
#8645=ADVANCED_FACE('',(#1228),#146,.T.);
#8646=ADVANCED_FACE('',(#1229),#147,.T.);
#8647=ADVANCED_FACE('',(#1230),#867,.T.);
#8648=ADVANCED_FACE('',(#1231),#88,.T.);
#8649=ADVANCED_FACE('',(#1232),#89,.T.);
#8650=ADVANCED_FACE('',(#1233),#90,.T.);
#8651=ADVANCED_FACE('',(#1234),#8229,.T.);
#8652=ADVANCED_FACE('',(#1235),#148,.F.);
#8653=ADVANCED_FACE('',(#1236),#91,.T.);
#8654=ADVANCED_FACE('',(#1237),#8230,.T.);
#8655=ADVANCED_FACE('',(#1238),#149,.F.);
#8656=ADVANCED_FACE('',(#1239),#150,.F.);
#8657=ADVANCED_FACE('',(#1240),#151,.F.);
#8658=ADVANCED_FACE('',(#1241),#152,.F.);
#8659=ADVANCED_FACE('',(#1242),#153,.F.);
#8660=ADVANCED_FACE('',(#1243),#154,.F.);
#8661=ADVANCED_FACE('',(#1244),#868,.F.);
#8662=ADVANCED_FACE('',(#1245,#627,#628,#629,#630,#631,#632),#869,.T.);
#8663=ADVANCED_FACE('',(#1246),#155,.F.);
#8664=ADVANCED_FACE('',(#1247),#870,.F.);
#8807=CLOSED_SHELL('',(#8562,#8563,#8564,#8565,#8566,#8567,#8568,#8569,
#8570,#8571,#8572,#8573,#8574,#8575,#8576,#8577,#8578,#8579,#8580,#8581,
#8582,#8583,#8584,#8585,#8586,#8587,#8588,#8589,#8590,#8591,#8592,#8593,
#8594,#8595,#8596,#8597,#8598,#8599,#8600,#8601,#8602,#8603,#8604,#8605,
#8606,#8607,#8608,#8609,#8610,#8611,#8612,#8613,#8614,#8615,#8616,#8617,
#8618,#8619,#8620,#8621,#8622,#8623,#8624,#8625,#8626,#8627,#8628,#8629,
#8630,#8631,#8632,#8633,#8634,#8635,#8636,#8637,#8638,#8639,#8640,#8641,
#8642,#8643,#8644,#8645,#8646,#8647,#8648,#8649,#8650,#8651,#8652,#8653,
#8654,#8655,#8656,#8657,#8658,#8659,#8660,#8661,#8662,#8663,#8664));
#9198=AXIS2_PLACEMENT_3D('',#14305,#10556,#10557);
#9199=AXIS2_PLACEMENT_3D('',#14306,#10558,#10559);
#9200=AXIS2_PLACEMENT_3D('',#14333,#10560,#10561);
#9201=AXIS2_PLACEMENT_3D('',#14334,#10562,#10563);
#9202=AXIS2_PLACEMENT_3D('',#14357,#10564,#10565);
#9203=AXIS2_PLACEMENT_3D('',#14358,#10566,#10567);
#9204=AXIS2_PLACEMENT_3D('',#14381,#10568,#10569);
#9205=AXIS2_PLACEMENT_3D('',#14382,#10570,#10571);
#9206=AXIS2_PLACEMENT_3D('',#14409,#10572,#10573);
#9207=AXIS2_PLACEMENT_3D('',#14594,#10574,#10575);
#9208=AXIS2_PLACEMENT_3D('',#14608,#10578,#10579);
#9209=AXIS2_PLACEMENT_3D('',#14610,#10580,#10581);
#9210=AXIS2_PLACEMENT_3D('',#14612,#10582,#10583);
#9211=AXIS2_PLACEMENT_3D('',#14613,#10584,#10585);
#9212=AXIS2_PLACEMENT_3D('',#14622,#10590,#10591);
#9213=AXIS2_PLACEMENT_3D('',#14628,#10595,#10596);
#9214=AXIS2_PLACEMENT_3D('',#14634,#10600,#10601);
#9215=AXIS2_PLACEMENT_3D('',#14640,#10605,#10606);
#9216=AXIS2_PLACEMENT_3D('',#14646,#10610,#10611);
#9217=AXIS2_PLACEMENT_3D('',#14649,#10614,#10615);
#9218=AXIS2_PLACEMENT_3D('',#14651,#10616,#10617);
#9219=AXIS2_PLACEMENT_3D('',#14652,#10618,#10619);
#9220=AXIS2_PLACEMENT_3D('',#14661,#10624,#10625);
#9221=AXIS2_PLACEMENT_3D('',#14667,#10629,#10630);
#9222=AXIS2_PLACEMENT_3D('',#14673,#10634,#10635);
#9223=AXIS2_PLACEMENT_3D('',#14679,#10639,#10640);
#9224=AXIS2_PLACEMENT_3D('',#14685,#10644,#10645);
#9225=AXIS2_PLACEMENT_3D('',#14688,#10648,#10649);
#9226=AXIS2_PLACEMENT_3D('',#14690,#10650,#10651);
#9227=AXIS2_PLACEMENT_3D('',#14691,#10652,#10653);
#9228=AXIS2_PLACEMENT_3D('',#14693,#10654,#10655);
#9229=AXIS2_PLACEMENT_3D('',#14695,#10657,#10658);
#9230=AXIS2_PLACEMENT_3D('',#14697,#10659,#10660);
#9231=AXIS2_PLACEMENT_3D('',#14700,#10662,#10663);
#9232=AXIS2_PLACEMENT_3D('',#14701,#10664,#10665);
#9233=AXIS2_PLACEMENT_3D('',#14703,#10666,#10667);
#9234=AXIS2_PLACEMENT_3D('',#14706,#10669,#10670);
#9235=AXIS2_PLACEMENT_3D('',#14707,#10671,#10672);
#9236=AXIS2_PLACEMENT_3D('',#14709,#10673,#10674);
#9237=AXIS2_PLACEMENT_3D('',#14711,#10676,#10677);
#9238=AXIS2_PLACEMENT_3D('',#14714,#10679,#10680);
#9239=AXIS2_PLACEMENT_3D('',#14715,#10681,#10682);
#9240=AXIS2_PLACEMENT_3D('',#14718,#10684,#10685);
#9241=AXIS2_PLACEMENT_3D('',#14719,#10686,#10687);
#9242=AXIS2_PLACEMENT_3D('',#14728,#10692,#10693);
#9243=AXIS2_PLACEMENT_3D('',#14737,#10698,#10699);
#9244=AXIS2_PLACEMENT_3D('',#14746,#10704,#10705);
#9245=AXIS2_PLACEMENT_3D('',#14755,#10710,#10711);
#9246=AXIS2_PLACEMENT_3D('',#14764,#10716,#10717);
#9247=AXIS2_PLACEMENT_3D('',#14773,#10722,#10723);
#9248=AXIS2_PLACEMENT_3D('',#14782,#10728,#10729);
#9249=AXIS2_PLACEMENT_3D('',#14784,#10730,#10731);
#9250=AXIS2_PLACEMENT_3D('',#14785,#10732,#10733);
#9251=AXIS2_PLACEMENT_3D('',#14787,#10734,#10735);
#9252=AXIS2_PLACEMENT_3D('',#14788,#10736,#10737);
#9253=AXIS2_PLACEMENT_3D('',#14791,#10740,#10741);
#9254=AXIS2_PLACEMENT_3D('',#14794,#10744,#10745);
#9255=AXIS2_PLACEMENT_3D('',#14797,#10748,#10749);
#9256=AXIS2_PLACEMENT_3D('',#14803,#10753,#10754);
#9257=AXIS2_PLACEMENT_3D('',#14809,#10758,#10759);
#9258=AXIS2_PLACEMENT_3D('',#14854,#10761,#10762);
#9259=AXIS2_PLACEMENT_3D('',#14900,#10765,#10766);
#9260=AXIS2_PLACEMENT_3D('',#14978,#10770,#10771);
#9261=AXIS2_PLACEMENT_3D('',#15026,#10775,#10776);
#9262=AXIS2_PLACEMENT_3D('',#15042,#10780,#10781);
#9263=AXIS2_PLACEMENT_3D('',#15363,#10793,#10794);
#9264=AXIS2_PLACEMENT_3D('',#15365,#10796,#10797);
#9265=AXIS2_PLACEMENT_3D('',#15367,#10798,#10799);
#9266=AXIS2_PLACEMENT_3D('',#15369,#10801,#10802);
#9267=AXIS2_PLACEMENT_3D('',#15533,#10804,#10805);
#9268=AXIS2_PLACEMENT_3D('',#15534,#10806,#10807);
#9269=AXIS2_PLACEMENT_3D('',#15582,#10809,#10810);
#9270=AXIS2_PLACEMENT_3D('',#15700,#10812,#10813);
#9271=AXIS2_PLACEMENT_3D('',#15745,#10814,#10815);
#9272=AXIS2_PLACEMENT_3D('',#15837,#10817,#10818);
#9273=AXIS2_PLACEMENT_3D('',#15854,#10819,#10820);
#9274=AXIS2_PLACEMENT_3D('',#15974,#10822,#10823);
#9275=AXIS2_PLACEMENT_3D('',#15979,#10824,#10825);
#9276=AXIS2_PLACEMENT_3D('',#16031,#10827,#10828);
#9277=AXIS2_PLACEMENT_3D('',#16032,#10829,#10830);
#9278=AXIS2_PLACEMENT_3D('',#16033,#10831,#10832);
#9279=AXIS2_PLACEMENT_3D('',#16034,#10833,#10834);
#9280=AXIS2_PLACEMENT_3D('',#16035,#10835,#10836);
#9281=AXIS2_PLACEMENT_3D('',#16036,#10837,#10838);
#9282=AXIS2_PLACEMENT_3D('',#16038,#10839,#10840);
#9283=AXIS2_PLACEMENT_3D('',#16039,#10841,#10842);
#9284=AXIS2_PLACEMENT_3D('',#16040,#10843,#10844);
#9285=AXIS2_PLACEMENT_3D('',#16041,#10845,#10846);
#9286=AXIS2_PLACEMENT_3D('',#16042,#10847,#10848);
#9287=AXIS2_PLACEMENT_3D('',#16043,#10849,#10850);
#9288=AXIS2_PLACEMENT_3D('',#16064,#10851,#10852);
#9289=AXIS2_PLACEMENT_3D('',#16066,#10853,#10854);
#9290=AXIS2_PLACEMENT_3D('',#16067,#10855,#10856);
#9291=AXIS2_PLACEMENT_3D('',#16068,#10857,#10858);
#9292=AXIS2_PLACEMENT_3D('',#16158,#10860,#10861);
#9293=AXIS2_PLACEMENT_3D('',#16159,#10862,#10863);
#9294=AXIS2_PLACEMENT_3D('',#16162,#10864,#10865);
#9295=AXIS2_PLACEMENT_3D('',#16164,#10866,#10867);
#9296=AXIS2_PLACEMENT_3D('',#16165,#10868,#10869);
#9297=AXIS2_PLACEMENT_3D('',#16166,#10870,#10871);
#9298=AXIS2_PLACEMENT_3D('',#16169,#10872,#10873);
#9299=AXIS2_PLACEMENT_3D('',#16171,#10874,#10875);
#9300=AXIS2_PLACEMENT_3D('',#16172,#10876,#10877);
#9301=AXIS2_PLACEMENT_3D('',#16173,#10878,#10879);
#9302=AXIS2_PLACEMENT_3D('',#16176,#10880,#10881);
#9303=AXIS2_PLACEMENT_3D('',#16178,#10882,#10883);
#9304=AXIS2_PLACEMENT_3D('',#16179,#10884,#10885);
#9305=AXIS2_PLACEMENT_3D('',#16180,#10886,#10887);
#9306=AXIS2_PLACEMENT_3D('',#16211,#10890,#10891);
#9307=AXIS2_PLACEMENT_3D('',#16214,#10892,#10893);
#9308=AXIS2_PLACEMENT_3D('',#16216,#10894,#10895);
#9309=AXIS2_PLACEMENT_3D('',#16217,#10896,#10897);
#9310=AXIS2_PLACEMENT_3D('',#16218,#10898,#10899);
#9311=AXIS2_PLACEMENT_3D('',#16391,#10902,#10903);
#9312=AXIS2_PLACEMENT_3D('',#16392,#10904,#10905);
#9313=AXIS2_PLACEMENT_3D('',#16409,#10906,#10907);
#10556=DIRECTION('axis',(0.,0.,1.));
#10557=DIRECTION('refdir',(1.,0.,0.));
#10558=DIRECTION('center_axis',(0.,0.,-1.));
#10559=DIRECTION('ref_axis',(1.,0.,0.));
#10560=DIRECTION('center_axis',(0.,0.,1.));
#10561=DIRECTION('ref_axis',(1.,0.,0.));
#10562=DIRECTION('center_axis',(0.,0.,-1.));
#10563=DIRECTION('ref_axis',(1.,0.,0.));
#10564=DIRECTION('center_axis',(0.,0.,1.));
#10565=DIRECTION('ref_axis',(1.,0.,0.));
#10566=DIRECTION('center_axis',(0.,0.,-1.));
#10567=DIRECTION('ref_axis',(1.,0.,0.));
#10568=DIRECTION('center_axis',(0.,0.,1.));
#10569=DIRECTION('ref_axis',(1.,0.,0.));
#10570=DIRECTION('center_axis',(0.,0.,-1.));
#10571=DIRECTION('ref_axis',(1.,0.,0.));
#10572=DIRECTION('center_axis',(0.,0.,1.));
#10573=DIRECTION('ref_axis',(1.,0.,0.));
#10574=DIRECTION('center_axis',(4.10828654779316E-33,-1.13946463231163E-19,
1.));
#10575=DIRECTION('ref_axis',(1.,0.,-4.10828654779316E-33));
#10576=DIRECTION('',(0.,1.,1.13946463231163E-19));
#10577=DIRECTION('',(0.,-1.,-1.13946463231163E-19));
#10578=DIRECTION('center_axis',(4.10828654779316E-33,-1.13946463231163E-19,
1.));
#10579=DIRECTION('ref_axis',(1.,0.,0.));
#10580=DIRECTION('center_axis',(4.10828654779316E-33,-1.13946463231163E-19,
1.));
#10581=DIRECTION('ref_axis',(1.,0.,0.));
#10582=DIRECTION('center_axis',(4.10828654779316E-33,-1.13946463231163E-19,
1.));
#10583=DIRECTION('ref_axis',(1.,0.,0.));
#10584=DIRECTION('center_axis',(0.86602540378444,0.499999999999998,0.));
#10585=DIRECTION('ref_axis',(0.499999999999998,-0.86602540378444,0.));
#10586=DIRECTION('',(0.499999999999998,-0.86602540378444,-9.86805318295791E-20));
#10587=DIRECTION('',(0.,0.,-1.));
#10588=DIRECTION('',(0.499999999999998,-0.86602540378444,0.));
#10589=DIRECTION('',(0.,0.,-1.));
#10590=DIRECTION('center_axis',(1.60246890531964E-16,1.,0.));
#10591=DIRECTION('ref_axis',(1.,-1.60246890531964E-16,0.));
#10592=DIRECTION('',(1.,-1.60246890531964E-16,-4.12654611421307E-33));
#10593=DIRECTION('',(0.,0.,-1.));
#10594=DIRECTION('',(1.,-1.60246890531964E-16,0.));
#10595=DIRECTION('center_axis',(-0.86602540378444,0.499999999999998,0.));
#10596=DIRECTION('ref_axis',(0.499999999999998,0.86602540378444,0.));
#10597=DIRECTION('',(0.499999999999998,0.86602540378444,9.86805318295749E-20));
#10598=DIRECTION('',(0.,0.,-1.));
#10599=DIRECTION('',(0.499999999999998,0.86602540378444,0.));
#10600=DIRECTION('center_axis',(-0.86602540378444,-0.499999999999998,0.));
#10601=DIRECTION('ref_axis',(-0.499999999999998,0.86602540378444,0.));
#10602=DIRECTION('',(-0.499999999999998,0.86602540378444,9.86805318295791E-20));
#10603=DIRECTION('',(0.,0.,-1.));
#10604=DIRECTION('',(-0.499999999999998,0.86602540378444,0.));
#10605=DIRECTION('center_axis',(-1.60246890531964E-16,-1.,0.));
#10606=DIRECTION('ref_axis',(-1.,1.60246890531964E-16,0.));
#10607=DIRECTION('',(-1.,1.60246890531964E-16,4.12654611421307E-33));
#10608=DIRECTION('',(0.,0.,-1.));
#10609=DIRECTION('',(-1.,1.60246890531964E-16,0.));
#10610=DIRECTION('center_axis',(0.86602540378444,-0.499999999999998,0.));
#10611=DIRECTION('ref_axis',(-0.499999999999998,-0.86602540378444,0.));
#10612=DIRECTION('',(-0.499999999999998,-0.86602540378444,-9.86805318295749E-20));
#10613=DIRECTION('',(-0.499999999999998,-0.86602540378444,0.));
#10614=DIRECTION('center_axis',(0.,0.,-1.));
#10615=DIRECTION('ref_axis',(-1.,0.,0.));
#10616=DIRECTION('center_axis',(0.,0.,1.));
#10617=DIRECTION('ref_axis',(1.,0.,0.));
#10618=DIRECTION('center_axis',(0.866025403784439,0.5,0.));
#10619=DIRECTION('ref_axis',(0.5,-0.866025403784439,0.));
#10620=DIRECTION('',(0.5,-0.866025403784439,-9.86805318295789E-20));
#10621=DIRECTION('',(0.,0.,-1.));
#10622=DIRECTION('',(0.5,-0.866025403784439,0.));
#10623=DIRECTION('',(0.,0.,-1.));
#10624=DIRECTION('center_axis',(1.60246890531964E-16,1.,0.));
#10625=DIRECTION('ref_axis',(1.,-1.60246890531964E-16,0.));
#10626=DIRECTION('',(1.,-1.60246890531964E-16,-4.12654611421307E-33));
#10627=DIRECTION('',(0.,0.,-1.));
#10628=DIRECTION('',(1.,-1.60246890531964E-16,0.));
#10629=DIRECTION('center_axis',(-0.866025403784438,0.5,0.));
#10630=DIRECTION('ref_axis',(0.5,0.866025403784438,0.));
#10631=DIRECTION('',(0.5,0.866025403784438,9.86805318295748E-20));
#10632=DIRECTION('',(0.,0.,-1.));
#10633=DIRECTION('',(0.5,0.866025403784438,0.));
#10634=DIRECTION('center_axis',(-0.866025403784439,-0.499999999999999,0.));
#10635=DIRECTION('ref_axis',(-0.499999999999999,0.866025403784439,0.));
#10636=DIRECTION('',(-0.499999999999999,0.866025403784439,9.8680531829579E-20));
#10637=DIRECTION('',(0.,0.,-1.));
#10638=DIRECTION('',(-0.499999999999999,0.866025403784439,0.));
#10639=DIRECTION('center_axis',(-1.60246890531964E-16,-1.,0.));
#10640=DIRECTION('ref_axis',(-1.,1.60246890531964E-16,0.));
#10641=DIRECTION('',(-1.,1.60246890531964E-16,4.12654611421307E-33));
#10642=DIRECTION('',(0.,0.,-1.));
#10643=DIRECTION('',(-1.,1.60246890531964E-16,0.));
#10644=DIRECTION('center_axis',(0.866025403784439,-0.5,0.));
#10645=DIRECTION('ref_axis',(-0.5,-0.866025403784439,0.));
#10646=DIRECTION('',(-0.5,-0.866025403784439,-9.86805318295748E-20));
#10647=DIRECTION('',(-0.5,-0.866025403784439,0.));
#10648=DIRECTION('center_axis',(0.,0.,-1.));
#10649=DIRECTION('ref_axis',(-1.,0.,0.));
#10650=DIRECTION('center_axis',(0.,0.,1.));
#10651=DIRECTION('ref_axis',(1.,0.,0.));
#10652=DIRECTION('center_axis',(0.,0.,-1.));
#10653=DIRECTION('ref_axis',(1.,0.,0.));
#10654=DIRECTION('center_axis',(-4.10828654779316E-33,1.13946463231163E-19,
-1.));
#10655=DIRECTION('ref_axis',(1.,0.,0.));
#10656=DIRECTION('',(0.,0.,-1.));
#10657=DIRECTION('center_axis',(0.,0.,-1.));
#10658=DIRECTION('ref_axis',(1.,0.,0.));
#10659=DIRECTION('center_axis',(-4.10828654779316E-33,1.13946463231163E-19,
-1.));
#10660=DIRECTION('ref_axis',(1.,0.,0.));
#10661=DIRECTION('',(0.,0.,-1.));
#10662=DIRECTION('center_axis',(4.10828654779316E-33,-1.13946463231163E-19,
1.));
#10663=DIRECTION('ref_axis',(1.,0.,0.));
#10664=DIRECTION('center_axis',(0.,0.,-1.));
#10665=DIRECTION('ref_axis',(1.,0.,0.));
#10666=DIRECTION('center_axis',(-4.10828654779316E-33,1.13946463231163E-19,
-1.));
#10667=DIRECTION('ref_axis',(1.,0.,0.));
#10668=DIRECTION('',(0.,0.,-1.));
#10669=DIRECTION('center_axis',(4.10828654779316E-33,-1.13946463231163E-19,
1.));
#10670=DIRECTION('ref_axis',(1.,0.,0.));
#10671=DIRECTION('center_axis',(0.,0.,-1.));
#10672=DIRECTION('ref_axis',(1.,0.,0.));
#10673=DIRECTION('center_axis',(-4.10828654779316E-33,1.13946463231163E-19,
-1.));
#10674=DIRECTION('ref_axis',(1.,0.,0.));
#10675=DIRECTION('',(0.,0.,-1.));
#10676=DIRECTION('center_axis',(0.,0.,-1.));
#10677=DIRECTION('ref_axis',(1.,0.,0.));
#10678=DIRECTION('',(0.,0.,-1.));
#10679=DIRECTION('center_axis',(0.,0.,1.));
#10680=DIRECTION('ref_axis',(1.,0.,0.));
#10681=DIRECTION('center_axis',(0.,0.,-1.));
#10682=DIRECTION('ref_axis',(1.,0.,0.));
#10683=DIRECTION('',(0.,0.,-1.));
#10684=DIRECTION('center_axis',(0.,0.,1.));
#10685=DIRECTION('ref_axis',(1.,0.,0.));
#10686=DIRECTION('center_axis',(0.,-1.,0.));
#10687=DIRECTION('ref_axis',(-1.,0.,0.));
#10688=DIRECTION('',(0.0523359562429438,0.,0.998629534754574));
#10689=DIRECTION('',(1.,0.,0.));
#10690=DIRECTION('',(-0.0523359562429438,0.,-0.998629534754574));
#10691=DIRECTION('',(1.,0.,0.));
#10692=DIRECTION('center_axis',(0.,-1.,0.));
#10693=DIRECTION('ref_axis',(-1.,0.,0.));
#10694=DIRECTION('',(0.,0.,-1.));
#10695=DIRECTION('',(1.,0.,0.));
#10696=DIRECTION('',(0.,0.,1.));
#10697=DIRECTION('',(1.,0.,0.));
#10698=DIRECTION('center_axis',(0.,-1.,0.));
#10699=DIRECTION('ref_axis',(-1.,0.,0.));
#10700=DIRECTION('',(0.,0.,-1.));
#10701=DIRECTION('',(1.,0.,0.));
#10702=DIRECTION('',(0.,0.,1.));
#10703=DIRECTION('',(1.,0.,0.));
#10704=DIRECTION('center_axis',(0.,-1.,0.));
#10705=DIRECTION('ref_axis',(-1.,0.,0.));
#10706=DIRECTION('',(0.,0.,-1.));
#10707=DIRECTION('',(1.,0.,0.));
#10708=DIRECTION('',(0.,0.,1.));
#10709=DIRECTION('',(1.,0.,0.));
#10710=DIRECTION('center_axis',(0.,1.,0.));
#10711=DIRECTION('ref_axis',(1.,0.,0.));
#10712=DIRECTION('',(-0.0523359562429438,0.,-0.998629534754574));
#10713=DIRECTION('',(-1.,0.,0.));
#10714=DIRECTION('',(0.0523359562429438,0.,0.998629534754574));
#10715=DIRECTION('',(-1.,0.,0.));
#10716=DIRECTION('center_axis',(0.,1.,0.));
#10717=DIRECTION('ref_axis',(1.,0.,0.));
#10718=DIRECTION('',(0.,0.,1.));
#10719=DIRECTION('',(-1.,0.,0.));
#10720=DIRECTION('',(0.,0.,-1.));
#10721=DIRECTION('',(-1.,0.,0.));
#10722=DIRECTION('center_axis',(0.,1.,0.));
#10723=DIRECTION('ref_axis',(1.,0.,0.));
#10724=DIRECTION('',(0.,0.,1.));
#10725=DIRECTION('',(-1.,0.,0.));
#10726=DIRECTION('',(0.,0.,-1.));
#10727=DIRECTION('',(-1.,0.,0.));
#10728=DIRECTION('center_axis',(0.,0.,1.));
#10729=DIRECTION('ref_axis',(1.,0.,0.));
#10730=DIRECTION('center_axis',(0.,0.,1.));
#10731=DIRECTION('ref_axis',(1.,0.,0.));
#10732=DIRECTION('center_axis',(0.,0.,1.));
#10733=DIRECTION('ref_axis',(1.,0.,0.));
#10734=DIRECTION('center_axis',(0.,0.,1.));
#10735=DIRECTION('ref_axis',(1.,0.,0.));
#10736=DIRECTION('center_axis',(0.,0.,1.));
#10737=DIRECTION('ref_axis',(1.,0.,0.));
#10738=DIRECTION('',(0.,1.,0.));
#10739=DIRECTION('',(0.,-1.,0.));
#10740=DIRECTION('center_axis',(0.,0.,1.));
#10741=DIRECTION('ref_axis',(1.,0.,0.));
#10742=DIRECTION('',(0.,-1.,0.));
#10743=DIRECTION('',(0.,1.,0.));
#10744=DIRECTION('center_axis',(0.,0.,1.));
#10745=DIRECTION('ref_axis',(1.,0.,0.));
#10746=DIRECTION('',(0.,-1.,0.));
#10747=DIRECTION('',(0.,1.,0.));
#10748=DIRECTION('center_axis',(0.,0.,1.));
#10749=DIRECTION('ref_axis',(1.,0.,0.));
#10750=DIRECTION('',(0.,-1.,0.));
#10751=DIRECTION('',(-1.,0.,0.));
#10752=DIRECTION('',(0.,1.,0.));
#10753=DIRECTION('center_axis',(0.,1.,0.));
#10754=DIRECTION('ref_axis',(1.,0.,0.));
#10755=DIRECTION('',(0.,0.,1.));
#10756=DIRECTION('',(-1.,0.,0.));
#10757=DIRECTION('',(0.,0.,-1.));
#10758=DIRECTION('center_axis',(-1.,0.,0.));
#10759=DIRECTION('ref_axis',(0.,-1.,0.));
#10760=DIRECTION('',(0.,-1.,0.));
#10761=DIRECTION('center_axis',(1.,0.,0.));
#10762=DIRECTION('ref_axis',(0.,1.,0.));
#10763=DIRECTION('',(0.,1.,0.));
#10764=DIRECTION('',(0.,1.,0.));
#10765=DIRECTION('center_axis',(1.,0.,0.));
#10766=DIRECTION('ref_axis',(0.,1.,0.));
#10767=DIRECTION('',(0.,1.,0.));
#10768=DIRECTION('',(0.,1.,1.13946463231163E-19));
#10769=DIRECTION('',(0.,1.,0.));
#10770=DIRECTION('center_axis',(1.,0.,0.));
#10771=DIRECTION('ref_axis',(0.,1.,0.));
#10772=DIRECTION('',(0.,1.,0.));
#10773=DIRECTION('',(0.,1.,1.13946463231163E-19));
#10774=DIRECTION('',(0.,1.,0.));
#10775=DIRECTION('center_axis',(0.998629534754574,0.,-0.0523359562429438));
#10776=DIRECTION('ref_axis',(-0.0523359562429438,0.,-0.998629534754574));
#10777=DIRECTION('',(0.,-1.,0.));
#10778=DIRECTION('',(-5.97168109510197E-21,-1.,-1.13946463231163E-19));
#10779=DIRECTION('',(0.,-1.,0.));
#10780=DIRECTION('center_axis',(0.,0.,1.));
#10781=DIRECTION('ref_axis',(1.,0.,0.));
#10782=DIRECTION('',(0.,-1.,0.));
#10783=DIRECTION('',(0.,-1.,0.));
#10784=DIRECTION('',(0.,-1.,0.));
#10785=DIRECTION('',(0.,1.,0.));
#10786=DIRECTION('',(0.,-1.,0.));
#10787=DIRECTION('',(0.,1.,0.));
#10788=DIRECTION('',(0.,-1.,0.));
#10789=DIRECTION('',(0.,-1.,0.));
#10790=DIRECTION('',(0.,-1.,0.));
#10791=DIRECTION('',(0.,1.,0.));
#10792=DIRECTION('',(0.,1.,0.));
#10793=DIRECTION('center_axis',(0.,0.,1.));
#10794=DIRECTION('ref_axis',(1.,0.,0.));
#10795=DIRECTION('',(0.,0.,-1.));
#10796=DIRECTION('center_axis',(0.,0.,1.));
#10797=DIRECTION('ref_axis',(1.,0.,0.));
#10798=DIRECTION('center_axis',(4.10828654779316E-33,-1.13946463231163E-19,
1.));
#10799=DIRECTION('ref_axis',(1.,0.,0.));
#10800=DIRECTION('',(0.,0.,-1.));
#10801=DIRECTION('center_axis',(1.,0.,0.));
#10802=DIRECTION('ref_axis',(0.,1.,0.));
#10803=DIRECTION('',(0.,1.,1.13946463231163E-19));
#10804=DIRECTION('center_axis',(0.99852593895705,0.0542765992849681,9.38276897523041E-9));
#10805=DIRECTION('ref_axis',(0.0541946171271057,-0.99701772369063,0.0549418066794405));
#10806=DIRECTION('center_axis',(4.10828654779316E-33,-1.13946463231163E-19,
1.));
#10807=DIRECTION('ref_axis',(1.,0.,-4.10828654779316E-33));
#10808=DIRECTION('',(5.97168109510217E-21,-1.,-1.13946463231163E-19));
#10809=DIRECTION('center_axis',(-1.,0.,0.));
#10810=DIRECTION('ref_axis',(0.,-1.,0.));
#10811=DIRECTION('',(0.,-1.,-1.13946463231163E-19));
#10812=DIRECTION('center_axis',(4.10828654779316E-33,-1.13946463231163E-19,
1.));
#10813=DIRECTION('ref_axis',(1.,0.,-4.10828654779316E-33));
#10814=DIRECTION('center_axis',(-1.,0.,0.));
#10815=DIRECTION('ref_axis',(0.,-1.,0.));
#10816=DIRECTION('',(0.,-1.,-1.13946463231163E-19));
#10817=DIRECTION('center_axis',(4.10828654779316E-33,-1.13946463231163E-19,
1.));
#10818=DIRECTION('ref_axis',(1.,0.,-4.10828654779316E-33));
#10819=DIRECTION('center_axis',(-1.,0.,0.));
#10820=DIRECTION('ref_axis',(0.,-1.,0.));
#10821=DIRECTION('',(0.,-1.,-1.13946463231163E-19));
#10822=DIRECTION('center_axis',(-0.996961060527779,0.0779015005717205,0.));
#10823=DIRECTION('ref_axis',(0.,0.,1.));
#10824=DIRECTION('center_axis',(4.10828654779316E-33,-1.13946463231163E-19,
1.));
#10825=DIRECTION('ref_axis',(1.,0.,-4.10828654779316E-33));
#10826=DIRECTION('',(5.97168109510197E-21,1.,1.13946463231163E-19));
#10827=DIRECTION('center_axis',(-0.996961060527779,-0.0779015005717276,
-4.485055189269E-15));
#10828=DIRECTION('ref_axis',(-0.0777791112471086,0.995394757055134,0.0560329142626144));
#10829=DIRECTION('center_axis',(-0.377317868652411,-0.840644185582845,0.388521015186253));
#10830=DIRECTION('ref_axis',(-0.58566693710526,0.541587807512093,0.603056287203763));
#10831=DIRECTION('center_axis',(7.41164423166535E-16,1.,0.));
#10832=DIRECTION('ref_axis',(0.,0.,1.));
#10833=DIRECTION('center_axis',(0.0522650005536027,-0.0520548592672972,
0.997275619547472));
#10834=DIRECTION('ref_axis',(-0.998629534754574,7.40148683083438E-16,0.0523359562429445));
#10835=DIRECTION('center_axis',(0.376559988603802,-0.837471124372148,0.396036224133039));
#10836=DIRECTION('ref_axis',(0.577069986161316,0.546481578685729,0.606916893181374));
#10837=DIRECTION('center_axis',(0.998525938475037,-0.0542766081525538,0.));
#10838=DIRECTION('ref_axis',(0.,0.,1.));
#10839=DIRECTION('center_axis',(-0.0522648366634829,-0.0521149007022807,
0.997272492337641));
#10840=DIRECTION('ref_axis',(0.0541946171271058,0.99701772369063,0.0549418066794413));
#10841=DIRECTION('center_axis',(5.32220538281047E-11,1.,-1.01553728389566E-9));
#10842=DIRECTION('ref_axis',(0.998629534754574,0.,0.0523359562429456));
#10843=DIRECTION('center_axis',(0.37731786865241,-0.840644185582843,-0.388521015186259));
#10844=DIRECTION('ref_axis',(-0.585666937105255,-0.541587807512095,0.603056287203766));
#10845=DIRECTION('center_axis',(0.0522650005536027,0.0520548592672965,0.997275619547472));
#10846=DIRECTION('ref_axis',(-0.0777791112471059,-0.995394757055134,0.0560329142626137));
#10847=DIRECTION('center_axis',(0.,-1.,0.));
#10848=DIRECTION('ref_axis',(-0.998629534754574,0.,0.0523359562429439));
#10849=DIRECTION('center_axis',(5.97168109510197E-21,1.,1.13946463231163E-19));
#10850=DIRECTION('ref_axis',(-0.688354575693753,0.,0.725374371012288));
#10851=DIRECTION('center_axis',(-0.376559987018669,-0.837471124206646,-0.396036225990193));
#10852=DIRECTION('ref_axis',(0.577069983350267,-0.54648157893936,0.606916895625808));
#10853=DIRECTION('center_axis',(-0.0522648366634817,0.0521149007022785,
0.997272492337641));
#10854=DIRECTION('ref_axis',(0.998629534754574,0.,0.052335956242946));
#10855=DIRECTION('center_axis',(1.01693095242295E-9,-1.,0.));
#10856=DIRECTION('ref_axis',(0.,0.,1.));
#10857=DIRECTION('center_axis',(5.97168109510217E-21,-1.,-1.13946463231163E-19));
#10858=DIRECTION('ref_axis',(0.688354575693753,0.,0.725374371012289));
#10859=DIRECTION('',(-5.97168109510217E-21,1.,1.13946463231163E-19));
#10860=DIRECTION('center_axis',(-0.998629534754574,0.,-0.0523359562429455));
#10861=DIRECTION('ref_axis',(-0.0523359562429455,0.,0.998629534754574));
#10862=DIRECTION('center_axis',(-0.377317868652411,-0.840644185582845,0.388521015186254));
#10863=DIRECTION('ref_axis',(-0.585666937105261,0.541587807512092,0.603056287203763));
#10864=DIRECTION('center_axis',(7.41164423166535E-16,1.,0.));
#10865=DIRECTION('ref_axis',(0.,0.,1.));
#10866=DIRECTION('center_axis',(-0.996961060527779,-0.0779015005717276,
-4.485055189269E-15));
#10867=DIRECTION('ref_axis',(-0.0777791112471086,0.995394757055134,0.0560329142626144));
#10868=DIRECTION('center_axis',(0.0522650005536027,-0.0520548592672972,
0.997275619547472));
#10869=DIRECTION('ref_axis',(-0.998629534754574,7.40148683083438E-16,0.0523359562429445));
#10870=DIRECTION('center_axis',(0.376559988603802,-0.837471124372148,0.396036224133039));
#10871=DIRECTION('ref_axis',(0.577069986161311,0.546481578685732,0.606916893181376));
#10872=DIRECTION('center_axis',(0.998525938475037,-0.0542766081525538,0.));
#10873=DIRECTION('ref_axis',(0.,0.,1.));
#10874=DIRECTION('center_axis',(5.32220538281047E-11,1.,-1.01553728389566E-9));
#10875=DIRECTION('ref_axis',(0.998629534754574,0.,0.0523359562429456));
#10876=DIRECTION('center_axis',(-0.0522648366634829,-0.0521149007022807,
0.997272492337641));
#10877=DIRECTION('ref_axis',(0.0541946171271058,0.99701772369063,0.0549418066794413));
#10878=DIRECTION('center_axis',(0.37731786865241,-0.840644185582843,-0.388521015186259));
#10879=DIRECTION('ref_axis',(-0.585666937105255,-0.541587807512095,0.603056287203766));
#10880=DIRECTION('center_axis',(-0.996961060527779,0.0779015005717205,0.));
#10881=DIRECTION('ref_axis',(0.,0.,1.));
#10882=DIRECTION('center_axis',(0.,-1.,0.));
#10883=DIRECTION('ref_axis',(-0.998629534754574,0.,0.0523359562429439));
#10884=DIRECTION('center_axis',(0.0522650005536027,0.0520548592672965,0.997275619547472));
#10885=DIRECTION('ref_axis',(-0.0777791112471059,-0.995394757055134,0.0560329142626137));
#10886=DIRECTION('center_axis',(5.97168109510197E-21,1.,1.13946463231163E-19));
#10887=DIRECTION('ref_axis',(-0.688354575693753,0.,0.725374371012289));
#10888=DIRECTION('',(-5.97168109510197E-21,-1.,-1.13946463231163E-19));
#10889=DIRECTION('',(5.97168109510197E-21,1.,1.13946463231163E-19));
#10890=DIRECTION('center_axis',(-0.376559987018669,-0.837471124206646,-0.396036225990194));
#10891=DIRECTION('ref_axis',(0.577069983350267,-0.546481578939359,0.606916895625808));
#10892=DIRECTION('center_axis',(-0.0522648366634817,0.0521149007022785,
0.997272492337641));
#10893=DIRECTION('ref_axis',(0.998629534754574,0.,0.052335956242946));
#10894=DIRECTION('center_axis',(1.01693095242295E-9,-1.,0.));
#10895=DIRECTION('ref_axis',(0.,0.,1.));
#10896=DIRECTION('center_axis',(0.99852593895705,0.0542765992849681,9.38276897523041E-9));
#10897=DIRECTION('ref_axis',(0.0541946171271057,-0.99701772369063,0.0549418066794405));
#10898=DIRECTION('center_axis',(5.97168109510217E-21,-1.,-1.13946463231163E-19));
#10899=DIRECTION('ref_axis',(0.688354575693753,0.,0.725374371012289));
#10900=DIRECTION('',(-5.97168109510217E-21,1.,1.13946463231163E-19));
#10901=DIRECTION('',(5.97168109510217E-21,-1.,-1.13946463231163E-19));
#10902=DIRECTION('center_axis',(0.998629534754574,0.,-0.0523359562429438));
#10903=DIRECTION('ref_axis',(-0.0523359562429438,0.,-0.998629534754574));
#10904=DIRECTION('center_axis',(4.10828654779316E-33,-1.13946463231163E-19,
1.));
#10905=DIRECTION('ref_axis',(1.,0.,-4.10828654779316E-33));
#10906=DIRECTION('center_axis',(-0.998629534754574,0.,-0.0523359562429455));
#10907=DIRECTION('ref_axis',(-0.0523359562429455,0.,0.998629534754574));
#14305=CARTESIAN_POINT('',(0.,0.,0.));
#14306=CARTESIAN_POINT('Origin',(8.1,-1.,0.7));
#14307=CARTESIAN_POINT('',(7.94916965151797,-1.19937453693185,0.7));
#14308=CARTESIAN_POINT('',(8.26514540988519,-1.18768855477586,0.7));
#14309=CARTESIAN_POINT('Ctrl Pts',(7.94916965151797,-1.19937453693185,0.7));
#14310=CARTESIAN_POINT('Ctrl Pts',(7.97160858810976,-1.21634998764782,0.7));
#14311=CARTESIAN_POINT('Ctrl Pts',(7.99739856866269,-1.22989011121344,0.69528529300377));
#14312=CARTESIAN_POINT('Ctrl Pts',(8.03944443766207,-1.24298414277179,0.688517705185315));
#14313=CARTESIAN_POINT('Ctrl Pts',(8.05362924383607,-1.24609346022897,0.686388676887586));
#14314=CARTESIAN_POINT('Ctrl Pts',(8.075506183533,-1.24890990228851,0.684139035126277));
#14315=CARTESIAN_POINT('Ctrl Pts',(8.08297567221474,-1.24953307703463,0.683546226354886));
#14316=CARTESIAN_POINT('Ctrl Pts',(8.0940066533036,-1.24995288972095,0.68299521602547));
#14317=CARTESIAN_POINT('Ctrl Pts',(8.09752287926269,-1.25001251279495,0.68286729538075));
#14318=CARTESIAN_POINT('Ctrl Pts',(8.10293413375911,-1.249989933108,0.682747340264197));
#14319=CARTESIAN_POINT('Ctrl Pts',(8.10482478940148,-1.24996059450444,0.682719828470948));
#14320=CARTESIAN_POINT('Ctrl Pts',(8.10828546792054,-1.24986760009171,0.682696100760705));
#14321=CARTESIAN_POINT('Ctrl Pts',(8.10985478687837,-1.24981062779486,0.682695370268813));
#14322=CARTESIAN_POINT('Ctrl Pts',(8.11326464342549,-1.24965465239671,0.682715595753076));
#14323=CARTESIAN_POINT('Ctrl Pts',(8.11510409202247,-1.2495501177419,0.682740330911594));
#14324=CARTESIAN_POINT('Ctrl Pts',(8.12014207260669,-1.24920790966494,0.682845651127781));
#14325=CARTESIAN_POINT('Ctrl Pts',(8.12333423895876,-1.24892926854386,0.682953992816581));
#14326=CARTESIAN_POINT('Ctrl Pts',(8.139194120874,-1.2472372768871,0.683691668462565));
#14327=CARTESIAN_POINT('Ctrl Pts',(8.15164141295685,-1.2449338270761,0.684918799511701));
#14328=CARTESIAN_POINT('Ctrl Pts',(8.19196937649467,-1.23428099896052,0.690212518998986));
#14329=CARTESIAN_POINT('Ctrl Pts',(8.21811504697062,-1.22213176592155,0.695755006185672));
#14330=CARTESIAN_POINT('Ctrl Pts',(8.24962874265135,-1.20052913769617,0.699397421419897));
#14331=CARTESIAN_POINT('Ctrl Pts',(8.25758631484639,-1.19433973204149,0.7));
#14332=CARTESIAN_POINT('Ctrl Pts',(8.26514540988519,-1.18768855477586,0.7));
#14333=CARTESIAN_POINT('Origin',(8.1,-1.,0.7));
#14334=CARTESIAN_POINT('Origin',(2.7,1.,0.7));
#14335=CARTESIAN_POINT('',(2.8076286513348,1.22564590451442,0.7));
#14336=CARTESIAN_POINT('',(2.57739843082973,1.21787348447435,0.7));
#14337=CARTESIAN_POINT('Ctrl Pts',(2.80762864495888,1.22564590575571,0.7));
#14338=CARTESIAN_POINT('Ctrl Pts',(2.78743249310418,1.23527907171202,0.7));
#14339=CARTESIAN_POINT('Ctrl Pts',(2.76507271635938,1.24261561512899,0.698430289974852));
#14340=CARTESIAN_POINT('Ctrl Pts',(2.73219941643314,1.24807722603274,0.696876198609429));
#14341=CARTESIAN_POINT('Ctrl Pts',(2.72335305886828,1.24906618730719,0.696525251810408));
#14342=CARTESIAN_POINT('Ctrl Pts',(2.71018695034311,1.24982905432238,0.696188910804419));
#14343=CARTESIAN_POINT('Ctrl Pts',(2.70590779780308,1.24996687586326,0.696107915309552));
#14344=CARTESIAN_POINT('Ctrl Pts',(2.69921702211412,1.25001037316246,0.696030339680738));
#14345=CARTESIAN_POINT('Ctrl Pts',(2.69680890442544,1.24999123464332,0.696012302673685));
#14346=CARTESIAN_POINT('Ctrl Pts',(2.69234597975348,1.24989125947742,0.695997601992606));
#14347=CARTESIAN_POINT('Ctrl Pts',(2.69029169500035,1.24981988388707,0.69599819279703));
#14348=CARTESIAN_POINT('Ctrl Pts',(2.6857660481318,1.24960673159635,0.696015705561832));
#14349=CARTESIAN_POINT('Ctrl Pts',(2.68329599580702,1.24945360531346,0.696035938105249));
#14350=CARTESIAN_POINT('Ctrl Pts',(2.67625328071593,1.24891193026541,0.696123377063474));
#14351=CARTESIAN_POINT('Ctrl Pts',(2.67169109188753,1.24843439216159,0.696216059649547));
#14352=CARTESIAN_POINT('Ctrl Pts',(2.64765560351845,1.24524789167778,0.696873729305584));
#14353=CARTESIAN_POINT('Ctrl Pts',(2.62857598726268,1.24037162800668,0.698048768812303));
#14354=CARTESIAN_POINT('Ctrl Pts',(2.59902076831046,1.22902239593109,0.699541037747764));
#14355=CARTESIAN_POINT('Ctrl Pts',(2.58799157881597,1.22383445108162,0.7));
#14356=CARTESIAN_POINT('Ctrl Pts',(2.57739843082979,1.21787348447436,0.7));
#14357=CARTESIAN_POINT('Origin',(2.7,1.,0.7));
#14358=CARTESIAN_POINT('Origin',(2.7,-1.,0.7));
#14359=CARTESIAN_POINT('',(2.57739843082979,-1.21787348447436,0.7));
#14360=CARTESIAN_POINT('',(2.80762864495888,-1.22564590575571,0.7));
#14361=CARTESIAN_POINT('Ctrl Pts',(2.57739843082979,-1.21787348447436,0.7));
#14362=CARTESIAN_POINT('Ctrl Pts',(2.59689796709118,-1.22884624579732,0.7));
#14363=CARTESIAN_POINT('Ctrl Pts',(2.61871070177046,-1.23767364961455,0.698430520021629));
#14364=CARTESIAN_POINT('Ctrl Pts',(2.6511387549791,-1.24533993869645,0.696876447160353));
#14365=CARTESIAN_POINT('Ctrl Pts',(2.65989793055836,-1.24692336726652,0.696525471319567));
#14366=CARTESIAN_POINT('Ctrl Pts',(2.67298219502323,-1.24857266139659,0.696189053183015));
#14367=CARTESIAN_POINT('Ctrl Pts',(2.67724223626036,-1.24899884484677,0.696108027479433));
#14368=CARTESIAN_POINT('Ctrl Pts',(2.68391475503581,-1.24949361628703,0.696030400846995));
#14369=CARTESIAN_POINT('Ctrl Pts',(2.68631866330158,-1.24963697932539,0.69601234479389));
#14370=CARTESIAN_POINT('Ctrl Pts',(2.69077815115796,-1.24983831390468,0.695997608323079));
#14371=CARTESIAN_POINT('Ctrl Pts',(2.69283257145917,-1.24990568929416,0.695998182544699));
#14372=CARTESIAN_POINT('Ctrl Pts',(2.69736230434386,-1.24999833696454,0.696015659042177));
#14373=CARTESIAN_POINT('Ctrl Pts',(2.69983707579759,-1.25001219669429,0.696035872086962));
#14374=CARTESIAN_POINT('Ctrl Pts',(2.70690037992806,-1.24994687665095,0.696123257636812));
#14375=CARTESIAN_POINT('Ctrl Pts',(2.71148446565418,-1.24977820005943,0.696215908504701));
#14376=CARTESIAN_POINT('Ctrl Pts',(2.73568105999059,-1.24822038288304,0.696873447340259));
#14377=CARTESIAN_POINT('Ctrl Pts',(2.75504695022812,-1.24464213141243,0.698048515307351));
#14378=CARTESIAN_POINT('Ctrl Pts',(2.78530198112344,-1.2353118289445,0.699540950501024));
#14379=CARTESIAN_POINT('Ctrl Pts',(2.79665680001786,-1.23087925931356,0.7));
#14380=CARTESIAN_POINT('Ctrl Pts',(2.80762864495888,-1.22564590575571,0.7));
#14381=CARTESIAN_POINT('Origin',(2.7,-1.,0.7));
#14382=CARTESIAN_POINT('Origin',(8.1,1.,0.7));
#14383=CARTESIAN_POINT('',(8.26514540988519,1.18768855477586,0.7));
#14384=CARTESIAN_POINT('',(7.94916965249954,1.19937453719419,0.7));
#14385=CARTESIAN_POINT('Ctrl Pts',(8.26514540988519,1.18768855477586,0.7));
#14386=CARTESIAN_POINT('Ctrl Pts',(8.24402114884725,1.20627559516199,0.7));
#14387=CARTESIAN_POINT('Ctrl Pts',(8.21930102059268,1.22168408824046,0.695284768760077));
#14388=CARTESIAN_POINT('Ctrl Pts',(8.17833936508797,1.23784683595578,0.688517484674842));
#14389=CARTESIAN_POINT('Ctrl Pts',(8.16442627443898,1.24199461640617,0.686388979601913));
#14390=CARTESIAN_POINT('Ctrl Pts',(8.14282164862934,1.24641910835203,0.684139556285851));
#14391=CARTESIAN_POINT('Ctrl Pts',(8.13541969045672,1.24759243465272,0.683546718614312));
#14392=CARTESIAN_POINT('Ctrl Pts',(8.12445132655127,1.24882623938238,0.682995554842566));
#14393=CARTESIAN_POINT('Ctrl Pts',(8.12094947916695,1.24914555886372,0.68286756899844));
#14394=CARTESIAN_POINT('Ctrl Pts',(8.11555178799172,1.24952297970176,0.682747494033431));
#14395=CARTESIAN_POINT('Ctrl Pts',(8.11366421100955,1.24963346420394,0.682719937279798));
#14396=CARTESIAN_POINT('Ctrl Pts',(8.11020620287515,1.24979651712922,0.682696124556263));
#14397=CARTESIAN_POINT('Ctrl Pts',(8.10863696767328,1.24985569708818,0.682695355189016));
#14398=CARTESIAN_POINT('Ctrl Pts',(8.10522484403353,1.249952190393,0.682715496638402));
#14399=CARTESIAN_POINT('Ctrl Pts',(8.10338263267786,1.24998390529834,0.682740187713169));
#14400=CARTESIAN_POINT('Ctrl Pts',(8.09833277498968,1.25001501472208,0.682845394223802));
#14401=CARTESIAN_POINT('Ctrl Pts',(8.09512844909059,1.24997307323179,0.682953673497893));
#14402=CARTESIAN_POINT('Ctrl Pts',(8.07918314804204,1.24945780552822,0.683691186949858));
#14403=CARTESIAN_POINT('Ctrl Pts',(8.06659630270856,1.24808001426183,0.684918585227095));
#14404=CARTESIAN_POINT('Ctrl Pts',(8.02558960427868,1.24043495378573,0.69021260546313));
#14405=CARTESIAN_POINT('Ctrl Pts',(7.9986188553413,1.2302509517108,0.695754623970086));
#14406=CARTESIAN_POINT('Ctrl Pts',(7.96559475436581,1.21103543221342,0.69939729083119));
#14407=CARTESIAN_POINT('Ctrl Pts',(7.95720051358587,1.20545002552208,0.7));
#14408=CARTESIAN_POINT('Ctrl Pts',(7.94916965151797,1.19937453693185,0.7));
#14409=CARTESIAN_POINT('Origin',(8.1,1.,0.7));
#14410=CARTESIAN_POINT('Ctrl Pts',(1.1,1.14549341399196,0.7));
#14411=CARTESIAN_POINT('Ctrl Pts',(1.89984199608574,1.1957170361627,0.7));
#14412=CARTESIAN_POINT('Ctrl Pts',(2.70080437300401,1.2273695200909,0.7));
#14413=CARTESIAN_POINT('Ctrl Pts',(3.50204003610941,1.24374118183538,0.7));
#14414=CARTESIAN_POINT('Ctrl Pts',(1.09819048660397,1.17431102498992,0.7));
#14415=CARTESIAN_POINT('Ctrl Pts',(1.89847848223077,1.22458382597074,0.70000077422621));
#14416=CARTESIAN_POINT('Ctrl Pts',(2.69984520196781,1.25626413437997,0.699999727319846));
#14417=CARTESIAN_POINT('Ctrl Pts',(3.50144932661635,1.27265074030048,0.700000000000001));
#14418=CARTESIAN_POINT('Ctrl Pts',(1.09505363188407,1.22426736091617,0.676703190608825));
#14419=CARTESIAN_POINT('Ctrl Pts',(1.89610976425884,1.27462253270773,0.67666760713801));
#14420=CARTESIAN_POINT('Ctrl Pts',(2.69818680938115,1.3063522351595,0.67664530655333));
#14421=CARTESIAN_POINT('Ctrl Pts',(3.50042536655637,1.322763754511,0.676632802377821));
#14422=CARTESIAN_POINT('Ctrl Pts',(1.09381704710221,1.24396073223232,0.627109609335854));
#14423=CARTESIAN_POINT('Ctrl Pts',(1.89518106151152,1.29430885982199,0.62701751976321));
#14424=CARTESIAN_POINT('Ctrl Pts',(2.69753328610131,1.32603127467068,0.626959208652505));
#14425=CARTESIAN_POINT('Ctrl Pts',(3.50002334924346,1.34243864233338,0.626926882269943));
#14426=CARTESIAN_POINT('Ctrl Pts',(1.09374258853658,1.24514653057163,0.605486452199395));
#14427=CARTESIAN_POINT('Ctrl Pts',(1.89512529323683,1.29547288309274,0.605377720397184));
#14428=CARTESIAN_POINT('Ctrl Pts',(2.69749615303001,1.32718177535833,0.605308474776761));
#14429=CARTESIAN_POINT('Ctrl Pts',(3.5,1.34358136363184,0.605270327458635));
#14430=CARTESIAN_POINT('',(1.1,1.14549341399195,0.7));
#14431=CARTESIAN_POINT('Ctrl Pts',(1.1,1.14549341399196,0.7));
#14432=CARTESIAN_POINT('Ctrl Pts',(1.59210562457523,1.17639367564078,0.7));
#14433=CARTESIAN_POINT('Ctrl Pts',(2.08463535466703,1.20026407570248,0.7));
#14434=CARTESIAN_POINT('Ctrl Pts',(2.57739190516306,1.2178709162388,0.7));
#14435=CARTESIAN_POINT('',(1.1,1.24553911298206,0.605485603995113));
#14436=CARTESIAN_POINT('Ctrl Pts',(1.1,1.14549341399196,0.7));
#14437=CARTESIAN_POINT('Ctrl Pts',(1.1,1.15341616150799,0.7));
#14438=CARTESIAN_POINT('Ctrl Pts',(1.1000012416168,1.16127613060545,0.699006361583129));
#14439=CARTESIAN_POINT('Ctrl Pts',(1.10000231308998,1.16893252943985,0.697119293189023));
#14440=CARTESIAN_POINT('Ctrl Pts',(1.10000291357081,1.17322337016277,0.696061732044743));
#14441=CARTESIAN_POINT('Ctrl Pts',(1.10000345673767,1.17745032641463,0.694722535963768));
#14442=CARTESIAN_POINT('Ctrl Pts',(1.10000379529503,1.18158693416151,0.693112479763539));
#14443=CARTESIAN_POINT('Ctrl Pts',(1.1000044034764,1.18901789868739,0.690220189452084));
#14444=CARTESIAN_POINT('Ctrl Pts',(1.1000042334852,1.19607766167095,0.686488065947256));
#14445=CARTESIAN_POINT('Ctrl Pts',(1.10000339376692,1.2026196529327,0.681996646156542));
#14446=CARTESIAN_POINT('Ctrl Pts',(1.10000293249552,1.20621327895058,0.67952943359521));
#14447=CARTESIAN_POINT('Ctrl Pts',(1.10000228571683,1.20965039763183,0.676832226278619));
#14448=CARTESIAN_POINT('Ctrl Pts',(1.10000171524363,1.21290279159005,0.673912896410569));
#14449=CARTESIAN_POINT('Ctrl Pts',(1.10000115816795,1.2160788033717,0.671062126739188));
#14450=CARTESIAN_POINT('Ctrl Pts',(1.10000066850715,1.2190594221245,0.668016750164662));
#14451=CARTESIAN_POINT('Ctrl Pts',(1.10000067525152,1.22182202639256,0.664788091882127));
#14452=CARTESIAN_POINT('Ctrl Pts',(1.10000068775799,1.22694487635592,0.658801012170571));
#14453=CARTESIAN_POINT('Ctrl Pts',(1.10000222199399,1.23132099043293,0.652185071179834));
#14454=CARTESIAN_POINT('Ctrl Pts',(1.10000276904041,1.23488987417606,0.64510534613808));
#14455=CARTESIAN_POINT('Ctrl Pts',(1.10000282439334,1.23525099193115,0.644388983656765));
#14456=CARTESIAN_POINT('Ctrl Pts',(1.10000287212626,1.23560380546488,0.64366785367332));
#14457=CARTESIAN_POINT('Ctrl Pts',(1.10000291138002,1.23594822450451,0.642942116631622));
#14458=CARTESIAN_POINT('Ctrl Pts',(1.10000329911404,1.23935026814133,0.635773555081239));
#14459=CARTESIAN_POINT('Ctrl Pts',(1.10000258010782,1.24189771450306,0.628240464257889));
#14460=CARTESIAN_POINT('Ctrl Pts',(1.10000149084855,1.24353681278199,0.620511076118615));
#14461=CARTESIAN_POINT('Ctrl Pts',(1.10000079446814,1.24458471384188,0.615569557890241));
#14462=CARTESIAN_POINT('Ctrl Pts',(1.10000000111128,1.24526049271905,0.610547146027233));
#14463=CARTESIAN_POINT('Ctrl Pts',(1.09999999916631,1.24553911263843,0.605485603997432));
#14464=CARTESIAN_POINT('',(3.5,1.34358136363184,0.605270327458635));
#14465=CARTESIAN_POINT('Ctrl Pts',(3.5,1.34358136363184,0.605270327458635));
#14466=CARTESIAN_POINT('Ctrl Pts',(2.6995848679345,1.32722445934619,0.605308375488923));
#14467=CARTESIAN_POINT('Ctrl Pts',(1.89930203168261,1.29563783986497,0.605377360150118));
#14468=CARTESIAN_POINT('Ctrl Pts',(1.09999999916631,1.24553911263843,0.605485603997431));
#14469=CARTESIAN_POINT('',(3.5,1.24369946473792,0.7));
#14470=CARTESIAN_POINT('Ctrl Pts',(3.5,1.34358136363184,0.605270327458635));
#14471=CARTESIAN_POINT('Ctrl Pts',(3.5,1.34316359984937,0.613184373088104));
#14472=CARTESIAN_POINT('Ctrl Pts',(3.50000057901142,1.34177887744868,0.621008021569537));
#14473=CARTESIAN_POINT('Ctrl Pts',(3.50000082863025,1.33951086762262,0.628580534231506));
#14474=CARTESIAN_POINT('Ctrl Pts',(3.50000096811,1.33824356956914,0.632811834486987));
#14475=CARTESIAN_POINT('Ctrl Pts',(3.50000102536574,1.33669948631919,0.636964759527324));
#14476=CARTESIAN_POINT('Ctrl Pts',(3.50000098105742,1.334886463945,0.641009258704104));
#14477=CARTESIAN_POINT('Ctrl Pts',(3.50000090179773,1.3316432906201,0.648244145614236));
#14478=CARTESIAN_POINT('Ctrl Pts',(3.50000044940971,1.3275777080273,0.655054131048541));
#14479=CARTESIAN_POINT('Ctrl Pts',(3.50000027423476,1.32275302640998,0.661275670751788));
#14480=CARTESIAN_POINT('Ctrl Pts',(3.50000024156065,1.32185311357394,0.66243612938574));
#14481=CARTESIAN_POINT('Ctrl Pts',(3.50000022115524,1.32092666334894,0.663576045687695));
#14482=CARTESIAN_POINT('Ctrl Pts',(3.50000022069074,1.31997391848392,0.664694242102532));
#14483=CARTESIAN_POINT('Ctrl Pts',(3.50000021976176,1.31806844339147,0.666930617752677));
#14484=CARTESIAN_POINT('Ctrl Pts',(3.50000029790302,1.31605782519,0.669080165434128));
#14485=CARTESIAN_POINT('Ctrl Pts',(3.50000040488465,1.31394946763378,0.671139079687271));
#14486=CARTESIAN_POINT('Ctrl Pts',(3.50000069329649,1.3082655455861,0.6766897075128));
#14487=CARTESIAN_POINT('Ctrl Pts',(3.5000011432336,1.30193818666762,0.681521899278667));
#14488=CARTESIAN_POINT('Ctrl Pts',(3.50000129797765,1.29513115062548,0.68558123547136));
#14489=CARTESIAN_POINT('Ctrl Pts',(3.50000139624096,1.2908086457691,0.688158936000333));
#14490=CARTESIAN_POINT('Ctrl Pts',(3.50000139493488,1.28629176508013,0.690424313967808));
#14491=CARTESIAN_POINT('Ctrl Pts',(3.50000129141552,1.28161680488022,0.692354162840695));
#14492=CARTESIAN_POINT('Ctrl Pts',(3.50000112941005,1.27430059661786,0.695374333209024));
#14493=CARTESIAN_POINT('Ctrl Pts',(3.5000007162179,1.26668229982361,0.697540280949125));
#14494=CARTESIAN_POINT('Ctrl Pts',(3.50000038344698,1.25890895215876,0.698782355543395));
#14495=CARTESIAN_POINT('Ctrl Pts',(3.50000016866387,1.25389173534334,0.699584038140014));
#14496=CARTESIAN_POINT('Ctrl Pts',(3.4999999993056,1.24880933504677,0.69999999987784));
#14497=CARTESIAN_POINT('Ctrl Pts',(3.49999999991873,1.24369946470729,0.7));
#14498=CARTESIAN_POINT('Ctrl Pts',(2.80762377174497,1.22564400643366,0.7));
#14499=CARTESIAN_POINT('Ctrl Pts',(3.03837960601223,1.23298334400942,0.7));
#14500=CARTESIAN_POINT('Ctrl Pts',(3.26917843294065,1.23897560812206,0.7));
#14501=CARTESIAN_POINT('Ctrl Pts',(3.49999999991873,1.24369946470729,0.7));
#14502=CARTESIAN_POINT('Ctrl Pts',(7.29709043526678,1.22049830417059,0.7));
#14503=CARTESIAN_POINT('Ctrl Pts',(8.19846709497879,1.19422430779862,0.7));
#14504=CARTESIAN_POINT('Ctrl Pts',(9.09944331332256,1.15544418981837,0.7));
#14505=CARTESIAN_POINT('Ctrl Pts',(10.,1.10900986674273,0.7));
#14506=CARTESIAN_POINT('Ctrl Pts',(7.29793284700474,1.24939875264889,0.7));
#14507=CARTESIAN_POINT('Ctrl Pts',(8.19957769811722,1.22310890030201,0.699999704549177));
#14508=CARTESIAN_POINT('Ctrl Pts',(9.10076698492607,1.18430758604571,0.700000491839571));
#14509=CARTESIAN_POINT('Ctrl Pts',(10.0014871213396,1.13785139984992,0.7));
#14510=CARTESIAN_POINT('Ctrl Pts',(7.29939288958794,1.29948813715084,0.676630595533454));
#14511=CARTESIAN_POINT('Ctrl Pts',(8.20149954052228,1.27317186922949,0.676644146017132));
#14512=CARTESIAN_POINT('Ctrl Pts',(9.10306300621911,1.23433322993607,0.676664155483857));
#14513=CARTESIAN_POINT('Ctrl Pts',(10.0040646682326,1.18784086746588,0.676686753673613));
#14514=CARTESIAN_POINT('Ctrl Pts',(7.29996660609513,1.31917051289423,0.626939603849942));
#14515=CARTESIAN_POINT('Ctrl Pts',(8.20225661204673,1.29285896783792,0.626974637782525));
#14516=CARTESIAN_POINT('Ctrl Pts',(9.10396596140606,1.25402923300358,0.627026849623412));
#14517=CARTESIAN_POINT('Ctrl Pts',(10.0050807923581,1.20754778500352,0.627085325222079));
#14518=CARTESIAN_POINT('Ctrl Pts',(7.29999999953093,1.32031613471704,0.605285370449856));
#14519=CARTESIAN_POINT('Ctrl Pts',(8.20230020786565,1.29401302889245,0.605326714446839));
#14520=CARTESIAN_POINT('Ctrl Pts',(9.10401978846669,1.25519559703033,0.605388684776982));
#14521=CARTESIAN_POINT('Ctrl Pts',(10.0051416645797,1.20872835322339,0.605457722909465));
#14522=CARTESIAN_POINT('',(7.29999999989017,1.22041345054104,0.7));
#14523=CARTESIAN_POINT('Ctrl Pts',(7.29999999978094,1.22041345055303,0.7));
#14524=CARTESIAN_POINT('Ctrl Pts',(7.51641201913776,1.21409884615949,0.7));
#14525=CARTESIAN_POINT('Ctrl Pts',(7.73280095443524,1.20706364503479,0.7));
#14526=CARTESIAN_POINT('Ctrl Pts',(7.94916654146952,1.19937499621344,0.7));
#14527=CARTESIAN_POINT('',(7.29999999953133,1.3203161347307,0.605285370449834));
#14528=CARTESIAN_POINT('Ctrl Pts',(7.29999999989087,1.22041345054982,0.7));
#14529=CARTESIAN_POINT('Ctrl Pts',(7.30000000079355,1.22832360919786,0.699999999740221));
#14530=CARTESIAN_POINT('Ctrl Pts',(7.29999941101664,1.23617007614594,0.699006006469939));
#14531=CARTESIAN_POINT('Ctrl Pts',(7.29999889581476,1.24381267896118,0.697118889344366));
#14532=CARTESIAN_POINT('Ctrl Pts',(7.29999860583198,1.24811433880851,0.696056720321257));
#14533=CARTESIAN_POINT('Ctrl Pts',(7.29999834128398,1.25235147078274,0.694710570513598));
#14534=CARTESIAN_POINT('Ctrl Pts',(7.29999817264931,1.25649739217805,0.693091458416622));
#14535=CARTESIAN_POINT('Ctrl Pts',(7.29999787070862,1.26392067210813,0.690192435210923));
#14536=CARTESIAN_POINT('Ctrl Pts',(7.29999793286912,1.27097116792553,0.686452948287278));
#14537=CARTESIAN_POINT('Ctrl Pts',(7.2999983123982,1.27750284616821,0.681954753865011));
#14538=CARTESIAN_POINT('Ctrl Pts',(7.2999985213788,1.28109939299731,0.679477906983553));
#14539=CARTESIAN_POINT('Ctrl Pts',(7.29999881895966,1.28453837241868,0.676770138671336));
#14540=CARTESIAN_POINT('Ctrl Pts',(7.29999908362886,1.28779148632494,0.673839551409954));
#14541=CARTESIAN_POINT('Ctrl Pts',(7.29999934163235,1.29096267037196,0.670982771155867));
#14542=CARTESIAN_POINT('Ctrl Pts',(7.29999957112158,1.2939379836903,0.667931525418885));
#14543=CARTESIAN_POINT('Ctrl Pts',(7.29999957127586,1.29669488996436,0.664697318929259));
#14544=CARTESIAN_POINT('Ctrl Pts',(7.29999957156178,1.30180432468448,0.658703293276094));
#14545=CARTESIAN_POINT('Ctrl Pts',(7.29999886995656,1.30616650855536,0.652082235935803));
#14546=CARTESIAN_POINT('Ctrl Pts',(7.29999863193158,1.30972187224872,0.644999691185358));
#14547=CARTESIAN_POINT('Ctrl Pts',(7.29999860759325,1.31008541227461,0.644275492840527));
#14548=CARTESIAN_POINT('Ctrl Pts',(7.29999858692673,1.31044047656777,0.643546449710686));
#14549=CARTESIAN_POINT('Ctrl Pts',(7.29999857034625,1.31078697300061,0.642812727646596));
#14550=CARTESIAN_POINT('Ctrl Pts',(7.29999840819729,1.31417553742296,0.635637287305567));
#14551=CARTESIAN_POINT('Ctrl Pts',(7.29999876577208,1.31670951795567,0.628098908385918));
#14552=CARTESIAN_POINT('Ctrl Pts',(7.29999928780719,1.3183355664444,0.620365998324013));
#14553=CARTESIAN_POINT('Ctrl Pts',(7.29999962266353,1.3193785856694,0.615405768714856));
#14554=CARTESIAN_POINT('Ctrl Pts',(7.3,1.32004717656055,0.610364828659741));
#14555=CARTESIAN_POINT('Ctrl Pts',(7.3,1.32031613470337,0.605285370449877));
#14556=CARTESIAN_POINT('',(10.,1.20899340483173,0.605457329065657));
#14557=CARTESIAN_POINT('Ctrl Pts',(9.99999999968202,1.20899340489109,0.605457329065633));
#14558=CARTESIAN_POINT('Ctrl Pts',(9.10058974048747,1.25534320916473,0.605388449123016));
#14559=CARTESIAN_POINT('Ctrl Pts',(8.20058408060299,1.29406305600824,0.605326635812744));
#14560=CARTESIAN_POINT('Ctrl Pts',(7.29999999953093,1.32031613471704,0.605285370449856));
#14561=CARTESIAN_POINT('',(9.99999999523418,1.1090098672342,0.7));
#14562=CARTESIAN_POINT('Ctrl Pts',(9.99999999968202,1.20899340489109,0.605457329065633));
#14563=CARTESIAN_POINT('Ctrl Pts',(9.99999999887489,1.20856043137698,0.613368813757176));
#14564=CARTESIAN_POINT('Ctrl Pts',(9.99999852309337,1.20715974444566,0.621187403383205));
#14565=CARTESIAN_POINT('Ctrl Pts',(9.99999786661901,1.20487567413208,0.628752957409046));
#14566=CARTESIAN_POINT('Ctrl Pts',(9.9999975031266,1.20361097553651,0.63294203403));
#14567=CARTESIAN_POINT('Ctrl Pts',(9.99999733971606,1.20207445367248,0.63705356322819));
#14568=CARTESIAN_POINT('Ctrl Pts',(9.99999742766416,1.20027388348257,0.64105842070465));
#14569=CARTESIAN_POINT('Ctrl Pts',(9.9999975865154,1.19702170610966,0.6482919664668));
#14570=CARTESIAN_POINT('Ctrl Pts',(9.99999868569093,1.19294650045069,0.655099368158521));
#14571=CARTESIAN_POINT('Ctrl Pts',(9.9999991134218,1.18811276085989,0.661317774786376));
#14572=CARTESIAN_POINT('Ctrl Pts',(9.99999919410111,1.18720101282252,0.662490701033652));
#14573=CARTESIAN_POINT('Ctrl Pts',(9.99999924414009,1.18626214680169,0.663642601192937));
#14574=CARTESIAN_POINT('Ctrl Pts',(9.99999924372355,1.18529642131707,0.664772262763739));
#14575=CARTESIAN_POINT('Ctrl Pts',(9.99999924291654,1.18342543943696,0.666960851926287));
#14576=CARTESIAN_POINT('Ctrl Pts',(9.99999905429896,1.18145367213587,0.669066014649603));
#14577=CARTESIAN_POINT('Ctrl Pts',(9.99999879621773,1.17938809187152,0.671084194359814));
#14578=CARTESIAN_POINT('Ctrl Pts',(9.99999808597787,1.17370361260899,0.676638227242868));
#14579=CARTESIAN_POINT('Ctrl Pts',(9.9999969699445,1.16737553754052,0.681473799108647));
#14580=CARTESIAN_POINT('Ctrl Pts',(9.99999660204079,1.16056788011185,0.685537070165577));
#14581=CARTESIAN_POINT('Ctrl Pts',(9.99999636768906,1.15623145667386,0.688125341392612));
#14582=CARTESIAN_POINT('Ctrl Pts',(9.99999638726733,1.15169947441128,0.690399565850749));
#14583=CARTESIAN_POINT('Ctrl Pts',(9.99999666360534,1.14700857532255,0.692336497939236));
#14584=CARTESIAN_POINT('Ctrl Pts',(9.99999709503399,1.13968497812548,0.695360504669253));
#14585=CARTESIAN_POINT('Ctrl Pts',(9.99999815490668,1.13205884654683,0.697530003145419));
#14586=CARTESIAN_POINT('Ctrl Pts',(9.99999900983214,1.12427739544825,0.698775573347137));
#14587=CARTESIAN_POINT('Ctrl Pts',(9.99999956314479,1.11924119569193,0.699581713521624));
#14588=CARTESIAN_POINT('Ctrl Pts',(10.,1.11413933950174,0.7));
#14589=CARTESIAN_POINT('Ctrl Pts',(10.,1.10900986674273,0.7));
#14590=CARTESIAN_POINT('Ctrl Pts',(8.26514054272776,1.18768929227839,0.7));
#14591=CARTESIAN_POINT('Ctrl Pts',(8.84359655063997,1.16547286645366,0.7));
#14592=CARTESIAN_POINT('Ctrl Pts',(9.42188471826001,1.13881853081542,0.7));
#14593=CARTESIAN_POINT('Ctrl Pts',(9.99999999522154,1.10900986698912,0.7));
#14594=CARTESIAN_POINT('Origin',(5.4,-8.11656130105013E-18,0.7));
#14595=CARTESIAN_POINT('',(7.3,-1.22041345053557,0.7));
#14596=CARTESIAN_POINT('Ctrl Pts',(7.94916654049851,-1.19937499624794,0.7));
#14597=CARTESIAN_POINT('Ctrl Pts',(7.73280095382446,-1.20706364505454,0.7));
#14598=CARTESIAN_POINT('Ctrl Pts',(7.51641201888728,-1.21409884616656,0.7));
#14599=CARTESIAN_POINT('Ctrl Pts',(7.29999999989085,-1.22041345054982,0.7));
#14600=CARTESIAN_POINT('',(7.3,-0.712777777777778,0.7));
#14601=CARTESIAN_POINT('',(10.,-1.10900986674244,0.7));
#14602=CARTESIAN_POINT('',(10.,0.653773457742722,0.7));
#14603=CARTESIAN_POINT('Ctrl Pts',(10.,-1.10900986674273,0.7));
#14604=CARTESIAN_POINT('Ctrl Pts',(9.42188472144661,-1.13881853066854,0.7));
#14605=CARTESIAN_POINT('Ctrl Pts',(8.84359655223373,-1.16547286639245,0.7));
#14606=CARTESIAN_POINT('Ctrl Pts',(8.26514054272776,-1.18768929227839,0.7));
#14607=CARTESIAN_POINT('',(7.95,-1.,0.7));
#14608=CARTESIAN_POINT('Origin',(8.1,-1.,0.7));
#14609=CARTESIAN_POINT('',(7.95,1.,0.7));
#14610=CARTESIAN_POINT('Origin',(8.1,1.,0.7));
#14611=CARTESIAN_POINT('',(8.4,-4.89858719658942E-17,0.7));
#14612=CARTESIAN_POINT('Origin',(8.8,0.,0.7));
#14613=CARTESIAN_POINT('Origin',(8.97320508075689,0.3,0.9));
#14614=CARTESIAN_POINT('',(8.97320508075689,0.3,0.9));
#14615=CARTESIAN_POINT('',(9.14641016151377,0.,0.9));
#14616=CARTESIAN_POINT('',(8.59150635094611,0.961121593216771,0.9));
#14617=CARTESIAN_POINT('',(8.97320508075689,0.3,0.6));
#14618=CARTESIAN_POINT('',(8.97320508075689,0.3,0.9));
#14619=CARTESIAN_POINT('',(9.14641016151377,0.,0.6));
#14620=CARTESIAN_POINT('',(9.14641016151377,0.,0.6));
#14621=CARTESIAN_POINT('',(9.14641016151377,0.,0.9));
#14622=CARTESIAN_POINT('Origin',(8.62679491924311,0.3,0.9));
#14623=CARTESIAN_POINT('',(8.62679491924311,0.3,0.9));
#14624=CARTESIAN_POINT('',(7.01339745962156,0.3,0.9));
#14625=CARTESIAN_POINT('',(8.62679491924311,0.3,0.6));
#14626=CARTESIAN_POINT('',(8.62679491924311,0.3,0.9));
#14627=CARTESIAN_POINT('',(8.97320508075689,0.3,0.6));
#14628=CARTESIAN_POINT('Origin',(8.45358983848623,5.55111512312578E-17,
0.9));
#14629=CARTESIAN_POINT('',(8.45358983848623,4.24230095489963E-17,0.9));
#14630=CARTESIAN_POINT('',(8.07189110867545,-0.661121593216771,0.9));
#14631=CARTESIAN_POINT('',(8.45358983848623,5.55111512312578E-17,0.6));
#14632=CARTESIAN_POINT('',(8.45358983848623,4.24230095489963E-17,0.9));
#14633=CARTESIAN_POINT('',(8.62679491924311,0.3,0.6));
#14634=CARTESIAN_POINT('Origin',(8.62679491924311,-0.3,0.9));
#14635=CARTESIAN_POINT('',(8.62679491924311,-0.3,0.9));
#14636=CARTESIAN_POINT('',(8.15849364905389,0.511121593216771,0.9));
#14637=CARTESIAN_POINT('',(8.62679491924311,-0.3,0.6));
#14638=CARTESIAN_POINT('',(8.62679491924311,-0.3,0.9));
#14639=CARTESIAN_POINT('',(8.45358983848623,4.24230095489963E-17,0.6));
#14640=CARTESIAN_POINT('Origin',(8.97320508075689,-0.3,0.9));
#14641=CARTESIAN_POINT('',(8.97320508075689,-0.3,0.9));
#14642=CARTESIAN_POINT('',(7.18660254037844,-0.3,0.9));
#14643=CARTESIAN_POINT('',(8.97320508075689,-0.3,0.6));
#14644=CARTESIAN_POINT('',(8.97320508075689,-0.3,0.9));
#14645=CARTESIAN_POINT('',(8.62679491924311,-0.3,0.6));
#14646=CARTESIAN_POINT('Origin',(9.14641016151377,0.,0.9));
#14647=CARTESIAN_POINT('',(8.67810889132456,-0.811121593216771,0.9));
#14648=CARTESIAN_POINT('',(8.97320508075689,-0.3,0.6));
#14649=CARTESIAN_POINT('Origin',(8.8,5.55111512312578E-17,0.6));
#14650=CARTESIAN_POINT('',(8.63,-2.0818995585505E-17,0.6));
#14651=CARTESIAN_POINT('Origin',(8.8,0.,0.6));
#14652=CARTESIAN_POINT('Origin',(2.17320508075689,0.3,0.9));
#14653=CARTESIAN_POINT('',(2.17320508075689,0.3,0.9));
#14654=CARTESIAN_POINT('',(2.34641016151378,0.,0.9));
#14655=CARTESIAN_POINT('',(2.64150635094611,-0.511121593216773,0.9));
#14656=CARTESIAN_POINT('',(2.17320508075689,0.3,0.6));
#14657=CARTESIAN_POINT('',(2.17320508075689,0.3,0.9));
#14658=CARTESIAN_POINT('',(2.34641016151378,0.,0.6));
#14659=CARTESIAN_POINT('',(2.34641016151378,0.,0.6));
#14660=CARTESIAN_POINT('',(2.34641016151378,0.,0.9));
#14661=CARTESIAN_POINT('Origin',(1.82679491924311,0.3,0.9));
#14662=CARTESIAN_POINT('',(1.82679491924311,0.3,0.9));
#14663=CARTESIAN_POINT('',(3.61339745962156,0.3,0.9));
#14664=CARTESIAN_POINT('',(1.82679491924311,0.3,0.6));
#14665=CARTESIAN_POINT('',(1.82679491924311,0.3,0.9));
#14666=CARTESIAN_POINT('',(2.17320508075689,0.3,0.6));
#14667=CARTESIAN_POINT('Origin',(1.65358983848622,5.55111512312578E-17,
0.9));
#14668=CARTESIAN_POINT('',(1.65358983848622,4.24230095489963E-17,0.9));
#14669=CARTESIAN_POINT('',(2.12189110867545,0.811121593216773,0.9));
#14670=CARTESIAN_POINT('',(1.65358983848622,5.55111512312578E-17,0.6));
#14671=CARTESIAN_POINT('',(1.65358983848622,4.24230095489963E-17,0.9));
#14672=CARTESIAN_POINT('',(1.82679491924311,0.3,0.6));
#14673=CARTESIAN_POINT('Origin',(1.82679491924311,-0.3,0.9));
#14674=CARTESIAN_POINT('',(1.82679491924311,-0.3,0.9));
#14675=CARTESIAN_POINT('',(2.20849364905389,-0.961121593216772,0.9));
#14676=CARTESIAN_POINT('',(1.82679491924311,-0.3,0.6));
#14677=CARTESIAN_POINT('',(1.82679491924311,-0.3,0.9));
#14678=CARTESIAN_POINT('',(1.65358983848622,4.24230095489963E-17,0.6));
#14679=CARTESIAN_POINT('Origin',(2.17320508075689,-0.3,0.9));
#14680=CARTESIAN_POINT('',(2.17320508075689,-0.3,0.9));
#14681=CARTESIAN_POINT('',(3.78660254037844,-0.3,0.9));
#14682=CARTESIAN_POINT('',(2.17320508075689,-0.3,0.6));
#14683=CARTESIAN_POINT('',(2.17320508075689,-0.3,0.9));
#14684=CARTESIAN_POINT('',(1.82679491924311,-0.3,0.6));
#14685=CARTESIAN_POINT('Origin',(2.34641016151378,0.,0.9));
#14686=CARTESIAN_POINT('',(2.72810889132455,0.661121593216773,0.9));
#14687=CARTESIAN_POINT('',(2.17320508075689,-0.3,0.6));
#14688=CARTESIAN_POINT('Origin',(2.,5.55111512312578E-17,0.6));
#14689=CARTESIAN_POINT('',(1.83,-2.0818995585505E-17,0.6));
#14690=CARTESIAN_POINT('Origin',(2.,0.,0.6));
#14691=CARTESIAN_POINT('Origin',(8.1,-1.,0.8));
#14692=CARTESIAN_POINT('',(7.95,-1.,0.9));
#14693=CARTESIAN_POINT('Origin',(8.1,-1.,0.9));
#14694=CARTESIAN_POINT('',(7.95,-1.,0.8));
#14695=CARTESIAN_POINT('Origin',(2.7,-1.,0.8));
#14696=CARTESIAN_POINT('',(2.55,-1.,0.9));
#14697=CARTESIAN_POINT('Origin',(2.7,-1.,0.9));
#14698=CARTESIAN_POINT('',(2.55,-1.,0.7));
#14699=CARTESIAN_POINT('',(2.55,-1.,0.8));
#14700=CARTESIAN_POINT('Origin',(2.7,-1.,0.7));
#14701=CARTESIAN_POINT('Origin',(2.7,1.,0.8));
#14702=CARTESIAN_POINT('',(2.55,1.,0.9));
#14703=CARTESIAN_POINT('Origin',(2.7,1.,0.9));
#14704=CARTESIAN_POINT('',(2.55,1.,0.7));
#14705=CARTESIAN_POINT('',(2.55,1.,0.8));
#14706=CARTESIAN_POINT('Origin',(2.7,1.,0.7));
#14707=CARTESIAN_POINT('Origin',(8.1,1.,0.8));
#14708=CARTESIAN_POINT('',(7.95,1.,0.9));
#14709=CARTESIAN_POINT('Origin',(8.1,1.,0.9));
#14710=CARTESIAN_POINT('',(7.95,1.,0.8));
#14711=CARTESIAN_POINT('Origin',(2.,0.,0.45));
#14712=CARTESIAN_POINT('',(1.83,-2.0818995585505E-17,0.32));
#14713=CARTESIAN_POINT('',(1.83,2.0818995585505E-17,0.45));
#14714=CARTESIAN_POINT('Origin',(2.,0.,0.32));
#14715=CARTESIAN_POINT('Origin',(8.8,0.,0.45));
#14716=CARTESIAN_POINT('',(8.63,-2.0818995585505E-17,0.32));
#14717=CARTESIAN_POINT('',(8.63,2.0818995585505E-17,0.45));
#14718=CARTESIAN_POINT('Origin',(8.8,0.,0.32));
#14719=CARTESIAN_POINT('Origin',(10.,-0.62,0.32));
#14720=CARTESIAN_POINT('',(0.200274469199584,-0.62,0.));
#14721=CARTESIAN_POINT('',(0.217044958570157,-0.62,0.32));
#14722=CARTESIAN_POINT('',(0.221783445591644,-0.62,0.410415718550007));
#14723=CARTESIAN_POINT('',(0.,-0.62,0.));
#14724=CARTESIAN_POINT('',(7.7,-0.62,0.));
#14725=CARTESIAN_POINT('',(0.0167704893705732,-0.62,0.32));
#14726=CARTESIAN_POINT('',(0.0220575386407278,-0.62,0.420882909798596));
#14727=CARTESIAN_POINT('',(-0.1,-0.62,0.32));
#14728=CARTESIAN_POINT('Origin',(10.,-0.62,0.32));
#14729=CARTESIAN_POINT('',(0.9,-0.62,0.32));
#14730=CARTESIAN_POINT('',(0.9,-0.62,0.));
#14731=CARTESIAN_POINT('',(0.9,-0.62,0.16));
#14732=CARTESIAN_POINT('',(1.1,-0.62,0.32));
#14733=CARTESIAN_POINT('',(-0.1,-0.62,0.32));
#14734=CARTESIAN_POINT('',(1.1,-0.62,0.));
#14735=CARTESIAN_POINT('',(1.1,-0.62,0.16));
#14736=CARTESIAN_POINT('',(7.7,-0.62,0.));
#14737=CARTESIAN_POINT('Origin',(10.,-0.62,0.32));
#14738=CARTESIAN_POINT('',(3.5,-0.62,0.32));
#14739=CARTESIAN_POINT('',(3.5,-0.62,0.));
#14740=CARTESIAN_POINT('',(3.5,-0.62,0.16));
#14741=CARTESIAN_POINT('',(3.7,-0.62,0.32));
#14742=CARTESIAN_POINT('',(-0.1,-0.62,0.32));
#14743=CARTESIAN_POINT('',(3.7,-0.62,0.));
#14744=CARTESIAN_POINT('',(3.7,-0.62,0.16));
#14745=CARTESIAN_POINT('',(7.7,-0.62,0.));
#14746=CARTESIAN_POINT('Origin',(10.,-0.62,0.32));
#14747=CARTESIAN_POINT('',(7.1,-0.62,0.32));
#14748=CARTESIAN_POINT('',(7.1,-0.62,0.));
#14749=CARTESIAN_POINT('',(7.1,-0.62,0.16));
#14750=CARTESIAN_POINT('',(7.3,-0.62,0.32));
#14751=CARTESIAN_POINT('',(-0.1,-0.62,0.32));
#14752=CARTESIAN_POINT('',(7.3,-0.62,0.));
#14753=CARTESIAN_POINT('',(7.3,-0.62,0.16));
#14754=CARTESIAN_POINT('',(7.7,-0.62,0.));
#14755=CARTESIAN_POINT('Origin',(-0.0999999999999996,0.62,0.32));
#14756=CARTESIAN_POINT('',(0.217044958570158,0.62,0.32));
#14757=CARTESIAN_POINT('',(0.200274469199584,0.62,0.));
#14758=CARTESIAN_POINT('',(0.207951231396534,0.62,0.146481348799182));
#14759=CARTESIAN_POINT('',(0.0167704893705736,0.62,0.32));
#14760=CARTESIAN_POINT('',(10.,0.62,0.32));
#14761=CARTESIAN_POINT('',(0.,0.62,0.));
#14762=CARTESIAN_POINT('',(0.00822532444561912,0.62,0.156948540047771));
#14763=CARTESIAN_POINT('',(2.65,0.62,0.));
#14764=CARTESIAN_POINT('Origin',(-0.0999999999999996,0.62,0.32));
#14765=CARTESIAN_POINT('',(0.9,0.62,0.));
#14766=CARTESIAN_POINT('',(0.9,0.62,0.32));
#14767=CARTESIAN_POINT('',(0.9,0.62,0.16));
#14768=CARTESIAN_POINT('',(1.1,0.62,0.));
#14769=CARTESIAN_POINT('',(2.65,0.62,0.));
#14770=CARTESIAN_POINT('',(1.1,0.62,0.32));
#14771=CARTESIAN_POINT('',(1.1,0.62,0.16));
#14772=CARTESIAN_POINT('',(10.,0.62,0.32));
#14773=CARTESIAN_POINT('Origin',(-0.0999999999999996,0.62,0.32));
#14774=CARTESIAN_POINT('',(3.5,0.62,0.));
#14775=CARTESIAN_POINT('',(3.5,0.62,0.32));
#14776=CARTESIAN_POINT('',(3.5,0.62,0.16));
#14777=CARTESIAN_POINT('',(3.7,0.62,0.));
#14778=CARTESIAN_POINT('',(2.65,0.62,0.));
#14779=CARTESIAN_POINT('',(3.7,0.62,0.32));
#14780=CARTESIAN_POINT('',(3.7,0.62,0.16));
#14781=CARTESIAN_POINT('',(10.,0.62,0.32));
#14782=CARTESIAN_POINT('Origin',(4.95,0.,0.32));
#14783=CARTESIAN_POINT('',(1.6,-4.89858719658941E-17,0.32));
#14784=CARTESIAN_POINT('Origin',(2.,0.,0.32));
#14785=CARTESIAN_POINT('Origin',(4.95,0.,0.32));
#14786=CARTESIAN_POINT('',(8.4,-4.89858719658942E-17,0.32));
#14787=CARTESIAN_POINT('Origin',(8.8,0.,0.32));
#14788=CARTESIAN_POINT('Origin',(4.95,0.,0.32));
#14789=CARTESIAN_POINT('',(0.217044958570157,-0.7,0.32));
#14790=CARTESIAN_POINT('',(0.0167704893705731,-0.7,0.32));
#14791=CARTESIAN_POINT('Origin',(4.95,0.,0.32));
#14792=CARTESIAN_POINT('',(0.9,0.671641708581009,0.32));
#14793=CARTESIAN_POINT('',(1.1,-0.671641708581009,0.32));
#14794=CARTESIAN_POINT('Origin',(4.95,0.,0.32));
#14795=CARTESIAN_POINT('',(3.5,0.723888888888889,0.32));
#14796=CARTESIAN_POINT('',(3.7,-0.723888888888889,0.32));
#14797=CARTESIAN_POINT('Origin',(4.95,0.,0.32));
#14798=CARTESIAN_POINT('',(7.1,0.62,0.32));
#14799=CARTESIAN_POINT('',(7.1,0.712777777777778,0.32));
#14800=CARTESIAN_POINT('',(7.3,0.62,0.32));
#14801=CARTESIAN_POINT('',(10.,0.62,0.32));
#14802=CARTESIAN_POINT('',(7.3,-0.712777777777778,0.32));
#14803=CARTESIAN_POINT('Origin',(-0.0999999999999996,0.62,0.32));
#14804=CARTESIAN_POINT('',(7.1,0.62,0.));
#14805=CARTESIAN_POINT('',(7.1,0.62,0.16));
#14806=CARTESIAN_POINT('',(7.3,0.62,0.));
#14807=CARTESIAN_POINT('',(2.65,0.62,0.));
#14808=CARTESIAN_POINT('',(7.3,0.62,0.16));
#14809=CARTESIAN_POINT('Origin',(10.,1.30754691548544,0.));
#14810=CARTESIAN_POINT('',(10.,1.24211782565704,0.));
#14811=CARTESIAN_POINT('',(10.,-1.24211782565704,0.));
#14812=CARTESIAN_POINT('',(10.,1.30754691548544,0.));
#14813=CARTESIAN_POINT('',(10.,-1.20899340483173,0.605457329065657));
#14814=CARTESIAN_POINT('Ctrl Pts',(10.,-1.20899340483173,0.605457329065657));
#14815=CARTESIAN_POINT('Ctrl Pts',(10.,-1.21451837038612,0.504502771559899));
#14816=CARTESIAN_POINT('Ctrl Pts',(10.,-1.22004249263249,0.403547366186347));
#14817=CARTESIAN_POINT('Ctrl Pts',(10.,-1.23108392958594,0.201728789021226));
#14818=CARTESIAN_POINT('Ctrl Pts',(10.,-1.23660133320922,0.100864020914724));
#14819=CARTESIAN_POINT('Ctrl Pts',(10.,-1.24211782565704,0.));
#14820=CARTESIAN_POINT('Ctrl Pts',(10.,-1.10900986674273,0.7));
#14821=CARTESIAN_POINT('Ctrl Pts',(10.,-1.11692706738765,0.7));
#14822=CARTESIAN_POINT('Ctrl Pts',(9.99999896020971,-1.12478097169818,0.699006158364426));
#14823=CARTESIAN_POINT('Ctrl Pts',(9.99999805494427,-1.13243115645175,0.697118998397561));
#14824=CARTESIAN_POINT('Ctrl Pts',(9.99999754769332,-1.13671781459207,0.696061558623929));
#14825=CARTESIAN_POINT('Ctrl Pts',(9.99999708556116,-1.14094056283945,0.694722610426682));
#14826=CARTESIAN_POINT('Ctrl Pts',(9.99999679002998,-1.14507302265453,0.693112977943955));
#14827=CARTESIAN_POINT('Ctrl Pts',(9.99999625879002,-1.15250143622127,0.690219540062595));
#14828=CARTESIAN_POINT('Ctrl Pts',(9.999996365957,-1.15955821040664,0.686485807665162));
#14829=CARTESIAN_POINT('Ctrl Pts',(9.99999703387985,-1.16609707610076,0.681992895329386));
#14830=CARTESIAN_POINT('Ctrl Pts',(9.99999740034986,-1.16968476316425,0.679527763880215));
#14831=CARTESIAN_POINT('Ctrl Pts',(9.99999792190556,-1.17311627083768,0.676833210412541));
#14832=CARTESIAN_POINT('Ctrl Pts',(9.99999838578331,-1.17636354905877,0.673917165661822));
#14833=CARTESIAN_POINT('Ctrl Pts',(9.99999884023993,-1.17954487655573,0.671060344436104));
#14834=CARTESIAN_POINT('Ctrl Pts',(9.99999924462882,-1.18253006594632,0.668008218820746));
#14835=CARTESIAN_POINT('Ctrl Pts',(9.99999924442301,-1.185296421281,0.664772262763763));
#14836=CARTESIAN_POINT('Ctrl Pts',(9.99999924404215,-1.19041578560695,0.658783864313737));
#14837=CARTESIAN_POINT('Ctrl Pts',(9.99999800949836,-1.19478865237554,0.652167294255586));
#14838=CARTESIAN_POINT('Ctrl Pts',(9.99999759228052,-1.19835462180986,0.645087621913151));
#14839=CARTESIAN_POINT('Ctrl Pts',(9.99999755030119,-1.19871341999785,0.644375284453517));
#14840=CARTESIAN_POINT('Ctrl Pts',(9.9999975145836,-1.19906401030029,0.643658239626438));
#14841=CARTESIAN_POINT('Ctrl Pts',(9.99999748581823,-1.19940630408966,0.642936645100882));
#14842=CARTESIAN_POINT('Ctrl Pts',(9.99999720003888,-1.20280693749908,0.635767720253638));
#14843=CARTESIAN_POINT('Ctrl Pts',(9.9999978299417,-1.20535324884233,0.628234501710241));
#14844=CARTESIAN_POINT('Ctrl Pts',(9.99999874867777,-1.20699142055415,0.62050509267719));
#14845=CARTESIAN_POINT('Ctrl Pts',(9.99999933690345,-1.20804026874419,0.615556297251186));
#14846=CARTESIAN_POINT('Ctrl Pts',(9.99999999916487,-1.20871598809812,0.61052641213707));
#14847=CARTESIAN_POINT('Ctrl Pts',(9.99999999968202,-1.20899340489109,0.605457329065633));
#14848=CARTESIAN_POINT('Ctrl Pts',(10.,1.24211782565704,0.));
#14849=CARTESIAN_POINT('Ctrl Pts',(10.,1.23660053043673,0.100878698875723));
#14850=CARTESIAN_POINT('Ctrl Pts',(10.,1.23108232376984,0.201758145268796));
#14851=CARTESIAN_POINT('Ctrl Pts',(10.,1.22004088630648,0.403576722396156));
#14852=CARTESIAN_POINT('Ctrl Pts',(10.,1.2145175671044,0.504517449470448));
#14853=CARTESIAN_POINT('Ctrl Pts',(10.,1.20899340483173,0.605457329065657));
#14854=CARTESIAN_POINT('Origin',(7.3,-1.42555555555556,0.));
#14855=CARTESIAN_POINT('',(7.3,1.35236351479115,0.));
#14856=CARTESIAN_POINT('',(7.3,-1.42555555555556,0.));
#14857=CARTESIAN_POINT('Ctrl Pts',(7.29999999953133,1.3203161347307,0.605285370449834));
#14858=CARTESIAN_POINT('Ctrl Pts',(7.29999999953133,1.32565322760551,0.504490726585133));
#14859=CARTESIAN_POINT('Ctrl Pts',(7.3,1.33099015509697,0.403695123734478));
#14860=CARTESIAN_POINT('Ctrl Pts',(7.3,1.34167258064689,0.201933969199042));
#14861=CARTESIAN_POINT('Ctrl Pts',(7.3,1.34701817868136,0.100966514951419));
#14862=CARTESIAN_POINT('Ctrl Pts',(7.3,1.35236351479115,0.));
#14863=CARTESIAN_POINT('',(7.29999999953133,-1.3203161347307,0.605285370449834));
#14864=CARTESIAN_POINT('Ctrl Pts',(7.3,-1.32031613470337,0.605285370449877));
#14865=CARTESIAN_POINT('Ctrl Pts',(7.3,-1.31989712778929,0.61319860217968));
#14866=CARTESIAN_POINT('Ctrl Pts',(7.29999916171872,-1.31851071739963,0.621020829077898));
#14867=CARTESIAN_POINT('Ctrl Pts',(7.29999878808195,-1.31624092632926,0.628591660945423));
#14868=CARTESIAN_POINT('Ctrl Pts',(7.29999857947278,-1.31497365483497,0.632818613610392));
#14869=CARTESIAN_POINT('Ctrl Pts',(7.29999848639856,-1.31343001415,0.636967235874856));
#14870=CARTESIAN_POINT('Ctrl Pts',(7.29999853830689,-1.31161789606625,0.641007613679984));
#14871=CARTESIAN_POINT('Ctrl Pts',(7.29999863125487,-1.30837308502546,0.648242386418365));
#14872=CARTESIAN_POINT('Ctrl Pts',(7.29999925734287,-1.30430566789097,0.655052076019481));
#14873=CARTESIAN_POINT('Ctrl Pts',(7.29999949821933,-1.29947941328181,0.661273460789274));
#14874=CARTESIAN_POINT('Ctrl Pts',(7.29999954322,-1.29857776968225,0.662435743389828));
#14875=CARTESIAN_POINT('Ctrl Pts',(7.29999957102613,-1.29764951297213,0.663577423078133));
#14876=CARTESIAN_POINT('Ctrl Pts',(7.2999995707084,-1.29669488998092,0.664697318929248));
#14877=CARTESIAN_POINT('Ctrl Pts',(7.29999957007561,-1.29479368240016,0.666927680549918));
#14878=CARTESIAN_POINT('Ctrl Pts',(7.29999945886743,-1.29278792931167,0.669071688571899));
#14879=CARTESIAN_POINT('Ctrl Pts',(7.29999930790078,-1.2906849717248,0.671125563583336));
#14880=CARTESIAN_POINT('Ctrl Pts',(7.29999889984047,-1.28500071247856,0.676677153447665));
#14881=CARTESIAN_POINT('Ctrl Pts',(7.29999826931494,-1.27867319504519,0.681510485910933));
#14882=CARTESIAN_POINT('Ctrl Pts',(7.29999806345125,-1.27186607945067,0.685571085769401));
#14883=CARTESIAN_POINT('Ctrl Pts',(7.29999793266427,-1.26754145993833,0.688150820039508));
#14884=CARTESIAN_POINT('Ctrl Pts',(7.29999794545359,-1.26302231037287,0.690417984675215));
#14885=CARTESIAN_POINT('Ctrl Pts',(7.29999810371711,-1.25834494218995,0.69234933099425));
#14886=CARTESIAN_POINT('Ctrl Pts',(7.29999835129001,-1.25102809722258,0.695370551698293));
#14887=CARTESIAN_POINT('Ctrl Pts',(7.29999895574222,-1.24340909242398,0.6975375590939));
#14888=CARTESIAN_POINT('Ctrl Pts',(7.29999944081525,-1.2356348173965,0.698780605629559));
#14889=CARTESIAN_POINT('Ctrl Pts',(7.29999975409932,-1.23061380764338,0.699583426311495));
#14890=CARTESIAN_POINT('Ctrl Pts',(7.30000000047446,-1.22552743956586,0.699999999832051));
#14891=CARTESIAN_POINT('Ctrl Pts',(7.29999999989087,-1.22041345054982,0.7));
#14892=CARTESIAN_POINT('',(7.3,-1.35236351479115,0.));
#14893=CARTESIAN_POINT('Ctrl Pts',(7.3,-1.35236351479115,0.));
#14894=CARTESIAN_POINT('Ctrl Pts',(7.3,-1.34701814920095,0.100967071798286));
#14895=CARTESIAN_POINT('Ctrl Pts',(7.3,-1.34167252169398,0.201935082699409));
#14896=CARTESIAN_POINT('Ctrl Pts',(7.3,-1.33099009614589,0.403696237111114));
#14897=CARTESIAN_POINT('Ctrl Pts',(7.29999999953133,-1.32565319812959,0.504491283257837));
#14898=CARTESIAN_POINT('Ctrl Pts',(7.29999999953133,-1.3203161347307,0.605285370449834));
#14899=CARTESIAN_POINT('',(7.3,-1.42555555555556,0.));
#14900=CARTESIAN_POINT('Origin',(3.7,-1.44777777777778,0.));
#14901=CARTESIAN_POINT('',(3.7,1.37924639543935,0.));
#14902=CARTESIAN_POINT('',(3.7,-1.44777777777778,0.));
#14903=CARTESIAN_POINT('',(3.7,1.34735368793805,0.605261457205193));
#14904=CARTESIAN_POINT('Ctrl Pts',(3.7,1.34735368793805,0.605261457205193));
#14905=CARTESIAN_POINT('Ctrl Pts',(3.7,1.35266395147774,0.504488703431434));
#14906=CARTESIAN_POINT('Ctrl Pts',(3.7,1.35797406404029,0.40371594170176));
#14907=CARTESIAN_POINT('Ctrl Pts',(3.7,1.36860496587027,0.201962122597264));
#14908=CARTESIAN_POINT('Ctrl Pts',(3.7,1.37392575452088,0.100981065191366));
#14909=CARTESIAN_POINT('Ctrl Pts',(3.7,1.37924639543935,0.));
#14910=CARTESIAN_POINT('',(3.7,1.24747724070879,0.7));
#14911=CARTESIAN_POINT('Ctrl Pts',(3.7,1.24747724070879,0.7));
#14912=CARTESIAN_POINT('Ctrl Pts',(3.7,1.25538532734776,0.7));
#14913=CARTESIAN_POINT('Ctrl Pts',(3.70000034866643,1.26322972530331,0.699006048248363));
#14914=CARTESIAN_POINT('Ctrl Pts',(3.70000065268588,1.27087026624727,0.697119044026295));
#14915=CARTESIAN_POINT('Ctrl Pts',(3.7000008238479,1.27517186762995,0.696056666371322));
#14916=CARTESIAN_POINT('Ctrl Pts',(3.70000097972585,1.27940891103121,0.694710185093394));
#14917=CARTESIAN_POINT('Ctrl Pts',(3.70000107833511,1.28355469746902,0.693090631030141));
#14918=CARTESIAN_POINT('Ctrl Pts',(3.70000125487464,1.29097687270382,0.690191153635441));
#14919=CARTESIAN_POINT('Ctrl Pts',(3.7000012145424,1.29802606517866,0.686451118058958));
#14920=CARTESIAN_POINT('Ctrl Pts',(3.70000098691147,1.3045562506385,0.681952404110064));
#14921=CARTESIAN_POINT('Ctrl Pts',(3.70000086156653,1.30815209635338,0.679475187900035));
#14922=CARTESIAN_POINT('Ctrl Pts',(3.70000068390876,1.31159030769532,0.676767042898431));
#14923=CARTESIAN_POINT('Ctrl Pts',(3.70000052608992,1.31484259178137,0.673836088143417));
#14924=CARTESIAN_POINT('Ctrl Pts',(3.70000037216713,1.31801458722906,0.670977489418868));
#14925=CARTESIAN_POINT('Ctrl Pts',(3.70000023558528,1.32099045552882,0.667924239810466));
#14926=CARTESIAN_POINT('Ctrl Pts',(3.70000023595245,1.32374763345498,0.664687876924229));
#14927=CARTESIAN_POINT('Ctrl Pts',(3.70000023663259,1.32885491153898,0.658692977181302));
#14928=CARTESIAN_POINT('Ctrl Pts',(3.70000065621025,1.33321474659758,0.652071180203097));
#14929=CARTESIAN_POINT('Ctrl Pts',(3.70000080093706,1.33676785491319,0.644988218508662));
#14930=CARTESIAN_POINT('Ctrl Pts',(3.70000081573428,1.33713113341147,0.644264039153811));
#14931=CARTESIAN_POINT('Ctrl Pts',(3.70000082835625,1.33748593861467,0.643535019157411));
#14932=CARTESIAN_POINT('Ctrl Pts',(3.70000083855542,1.33783217873901,0.642801324492746));
#14933=CARTESIAN_POINT('Ctrl Pts',(3.70000093832019,1.34121897990539,0.63562457699476));
#14934=CARTESIAN_POINT('Ctrl Pts',(3.70000072997693,1.34375116782692,0.628085030530103));
#14935=CARTESIAN_POINT('Ctrl Pts',(3.70000042189378,1.34537558692779,0.6203512574804));
#14936=CARTESIAN_POINT('Ctrl Pts',(3.70000022417294,1.3464181026242,0.615387895628485));
#14937=CARTESIAN_POINT('Ctrl Pts',(3.70000000036652,1.34708586836718,0.6103438638189));
#14938=CARTESIAN_POINT('Ctrl Pts',(3.69999999992214,1.34735368792773,0.6052614572053));
#14939=CARTESIAN_POINT('',(3.7,-1.24747724070944,0.7));
#14940=CARTESIAN_POINT('',(3.7,-0.723888888888889,0.7));
#14941=CARTESIAN_POINT('',(3.7,-1.34735368793805,0.605261457205193));
#14942=CARTESIAN_POINT('Ctrl Pts',(3.69999999992215,-1.34735368792773,0.6052614572053));
#14943=CARTESIAN_POINT('Ctrl Pts',(3.70000000061408,-1.34693666923469,0.613175212866596));
#14944=CARTESIAN_POINT('Ctrl Pts',(3.70000049671034,-1.34555248374866,0.620998392122869));
#14945=CARTESIAN_POINT('Ctrl Pts',(3.70000071566022,-1.34328499565267,0.628570462735333));
#14946=CARTESIAN_POINT('Ctrl Pts',(3.70000083807517,-1.34201724238155,0.632804009674372));
#14947=CARTESIAN_POINT('Ctrl Pts',(3.7000008913247,-1.34047237297042,0.63695909738719));
#14948=CARTESIAN_POINT('Ctrl Pts',(3.70000085837557,-1.33865827982058,0.641005656934072));
#14949=CARTESIAN_POINT('Ctrl Pts',(3.7000007994669,-1.33541492172585,0.648240369034365));
#14950=CARTESIAN_POINT('Ctrl Pts',(3.70000042420685,-1.33134915897915,0.655050234746405));
#14951=CARTESIAN_POINT('Ctrl Pts',(3.70000027984635,-1.32652447879733,0.661271863919233));
#14952=CARTESIAN_POINT('Ctrl Pts',(3.70000025294096,-1.32562527203035,0.662431429080655));
#14953=CARTESIAN_POINT('Ctrl Pts',(3.7000002362737,-1.32469957579387,0.663570491348455));
#14954=CARTESIAN_POINT('Ctrl Pts',(3.70000023630138,-1.32374763346102,0.664687876924223));
#14955=CARTESIAN_POINT('Ctrl Pts',(3.70000023635686,-1.32184039796576,0.666926581264246));
#14956=CARTESIAN_POINT('Ctrl Pts',(3.70000030283857,-1.31982784222224,0.669078323867587));
#14957=CARTESIAN_POINT('Ctrl Pts',(3.70000039320883,-1.31771738411303,0.671139279696989));
#14958=CARTESIAN_POINT('Ctrl Pts',(3.70000063660146,-1.3120333248939,0.676690015307994));
#14959=CARTESIAN_POINT('Ctrl Pts',(3.7000010126336,-1.30570602994251,0.681522474044465));
#14960=CARTESIAN_POINT('Ctrl Pts',(3.70000113724274,-1.29889910811053,0.685582059356066));
#14961=CARTESIAN_POINT('Ctrl Pts',(3.70000121634872,-1.29457784995583,0.688159217808216));
#14962=CARTESIAN_POINT('Ctrl Pts',(3.70000121058612,-1.2900623422215,0.690424215862126));
#14963=CARTESIAN_POINT('Ctrl Pts',(3.70000111831253,-1.28538881676413,0.692353818784707));
#14964=CARTESIAN_POINT('Ctrl Pts',(3.70000097388434,-1.27807373536961,0.695374066040565));
#14965=CARTESIAN_POINT('Ctrl Pts',(3.70000061691996,-1.27045659963863,0.697540160564298));
#14966=CARTESIAN_POINT('Ctrl Pts',(3.7000003304055,-1.26268427129293,0.698782316368755));
#14967=CARTESIAN_POINT('Ctrl Pts',(3.70000014548661,-1.25766794365683,0.699584014420239));
#14968=CARTESIAN_POINT('Ctrl Pts',(3.7,-1.25258637988459,0.7));
#14969=CARTESIAN_POINT('Ctrl Pts',(3.7,-1.24747724070879,0.7));
#14970=CARTESIAN_POINT('',(3.7,-1.37924639543935,0.));
#14971=CARTESIAN_POINT('Ctrl Pts',(3.7,-1.37924639543935,0.));
#14972=CARTESIAN_POINT('Ctrl Pts',(3.7,-1.37392574223662,0.100981298335747));
#14973=CARTESIAN_POINT('Ctrl Pts',(3.7,-1.36860494130098,0.201962588887634));
#14974=CARTESIAN_POINT('Ctrl Pts',(3.7,-1.35797403946962,0.403716407992068));
#14975=CARTESIAN_POINT('Ctrl Pts',(3.7,-1.3526639391921,0.504488936575732));
#14976=CARTESIAN_POINT('Ctrl Pts',(3.7,-1.34735368793805,0.605261457205193));
#14977=CARTESIAN_POINT('',(3.7,-1.44777777777778,0.));
#14978=CARTESIAN_POINT('Origin',(1.1,-1.34328341716202,0.));
#14979=CARTESIAN_POINT('',(1.1,1.27885335043294,0.));
#14980=CARTESIAN_POINT('',(1.1,-1.34328341716202,0.));
#14981=CARTESIAN_POINT('Ctrl Pts',(1.1,1.24553911298206,0.605485603995113));
#14982=CARTESIAN_POINT('Ctrl Pts',(1.1,1.25109559382646,0.504544105903265));
#14983=CARTESIAN_POINT('Ctrl Pts',(1.1,1.25665083308595,0.403601248768354));
#14984=CARTESIAN_POINT('Ctrl Pts',(1.1,1.26775551906787,0.201773573764085));
#14985=CARTESIAN_POINT('Ctrl Pts',(1.1,1.2733051088238,0.100886182270816));
#14986=CARTESIAN_POINT('Ctrl Pts',(1.1,1.27885335043294,0.));
#14987=CARTESIAN_POINT('',(1.1,-1.14549341399195,0.7));
#14988=CARTESIAN_POINT('',(1.1,-0.671641708581009,0.7));
#14989=CARTESIAN_POINT('',(1.1,-1.24553911298206,0.605485603995113));
#14990=CARTESIAN_POINT('Ctrl Pts',(1.09999999916631,-1.24553911263843,0.605485603997431));
#14991=CARTESIAN_POINT('Ctrl Pts',(1.10000000220634,-1.24510362317222,0.61339691285734));
#14992=CARTESIAN_POINT('Ctrl Pts',(1.10000177015643,-1.24370036622144,0.621215229994996));
#14993=CARTESIAN_POINT('Ctrl Pts',(1.10000252895322,-1.24141353486351,0.628780213666851));
#14994=CARTESIAN_POINT('Ctrl Pts',(1.10000294802756,-1.24015054543059,0.632958263090869));
#14995=CARTESIAN_POINT('Ctrl Pts',(1.10000312162076,-1.23861706177488,0.637059070655947));
#14996=CARTESIAN_POINT('Ctrl Pts',(1.10000299297862,-1.23682078380192,0.641053713130525));
#14997=CARTESIAN_POINT('Ctrl Pts',(1.10000275999609,-1.23356756237267,0.64828837095969));
#14998=CARTESIAN_POINT('Ctrl Pts',(1.10000138715103,-1.22949085733774,0.655096441442141));
#14999=CARTESIAN_POINT('Ctrl Pts',(1.10000084482056,-1.2246552743941,0.661315040399663));
#15000=CARTESIAN_POINT('Ctrl Pts',(1.10000074196669,-1.22373819809959,0.662494407966206));
#15001=CARTESIAN_POINT('Ctrl Pts',(1.1000006773267,-1.22279369438101,0.663652502541609));
#15002=CARTESIAN_POINT('Ctrl Pts',(1.10000067553493,-1.22182202641035,0.66478809188211));
#15003=CARTESIAN_POINT('Ctrl Pts',(1.10000067210542,-1.219962222636,0.666961646435043));
#15004=CARTESIAN_POINT('Ctrl Pts',(1.10000089707048,-1.21800293160495,0.669052796220007));
#15005=CARTESIAN_POINT('Ctrl Pts',(1.10000120920309,-1.21595100691259,0.671058078730413));
#15006=CARTESIAN_POINT('Ctrl Pts',(1.10000207391986,-1.21026645613745,0.676613414309409));
#15007=CARTESIAN_POINT('Ctrl Pts',(1.1000034579227,-1.20393786500476,0.681450029097565));
#15008=CARTESIAN_POINT('Ctrl Pts',(1.10000394126019,-1.19712964857754,0.685514663758263));
#15009=CARTESIAN_POINT('Ctrl Pts',(1.10000424974863,-1.19278432848208,0.688108902478585));
#15010=CARTESIAN_POINT('Ctrl Pts',(1.10000425197701,-1.18824265871575,0.690387991283085));
#15011=CARTESIAN_POINT('Ctrl Pts',(1.10000394032285,-1.18354156621637,0.692328715646671));
#15012=CARTESIAN_POINT('Ctrl Pts',(1.10000345443802,-1.17621232165581,0.695354404566264));
#15013=CARTESIAN_POINT('Ctrl Pts',(1.10000219938511,-1.16858027633095,0.697525330589554));
#15014=CARTESIAN_POINT('Ctrl Pts',(1.10000118192936,-1.16079305972554,0.698772417158578));
#15015=CARTESIAN_POINT('Ctrl Pts',(1.10000052251962,-1.15574619011492,0.699580649884844));
#15016=CARTESIAN_POINT('Ctrl Pts',(1.1,-1.15063354328712,0.7));
#15017=CARTESIAN_POINT('Ctrl Pts',(1.1,-1.14549341399196,0.7));
#15018=CARTESIAN_POINT('',(1.1,-1.27885335043294,0.));
#15019=CARTESIAN_POINT('Ctrl Pts',(1.1,-1.27885335043294,0.));
#15020=CARTESIAN_POINT('Ctrl Pts',(1.1,-1.27330503870861,0.100887457206881));
#15021=CARTESIAN_POINT('Ctrl Pts',(1.1,-1.26775537880223,0.201776123688554));
#15022=CARTESIAN_POINT('Ctrl Pts',(1.1,-1.25665069275548,0.403603798678134));
#15023=CARTESIAN_POINT('Ctrl Pts',(1.1,-1.25109552364596,0.504545380833391));
#15024=CARTESIAN_POINT('Ctrl Pts',(1.1,-1.24553911298206,0.605485603995113));
#15025=CARTESIAN_POINT('',(1.1,-1.34328341716202,0.));
#15026=CARTESIAN_POINT('Origin',(0.199725906950915,-1.4,-0.0104671912485888));
#15027=CARTESIAN_POINT('',(0.200274469199584,1.12301388185427,1.38777878078145E-17));
#15028=CARTESIAN_POINT('',(0.200274469199585,-0.7,0.));
#15029=CARTESIAN_POINT('',(0.231993417893744,1.09142177001972,0.605233595624295));
#15030=CARTESIAN_POINT('Ctrl Pts',(0.200274469199584,1.12301388185427,-2.97071395261028E-17));
#15031=CARTESIAN_POINT('Ctrl Pts',(0.210847451470635,1.11248294808,0.201744519910852));
#15032=CARTESIAN_POINT('Ctrl Pts',(0.22142043436526,1.101952242875,0.403489051720196));
#15033=CARTESIAN_POINT('Ctrl Pts',(0.231993417893744,1.09142177001972,0.605233595624295));
#15034=CARTESIAN_POINT('',(0.231993417893744,-1.09142177001972,0.605233595624295));
#15035=CARTESIAN_POINT('',(0.231993417893744,-0.7,0.605233595624295));
#15036=CARTESIAN_POINT('',(0.200274469199584,-1.12301388185427,-1.38777878078145E-17));
#15037=CARTESIAN_POINT('Ctrl Pts',(0.231993417893744,-1.09142177001972,
0.605233595624295));
#15038=CARTESIAN_POINT('Ctrl Pts',(0.22142043436526,-1.101952242875,0.403489051720196));
#15039=CARTESIAN_POINT('Ctrl Pts',(0.210847451470635,-1.11248294808,0.201744519910852));
#15040=CARTESIAN_POINT('Ctrl Pts',(0.200274469199584,-1.12301388185427,
-4.90059381963448E-17));
#15041=CARTESIAN_POINT('',(0.200274469199585,-0.7,0.));
#15042=CARTESIAN_POINT('Origin',(5.4,-1.11022302462516E-16,0.));
#15043=CARTESIAN_POINT('Ctrl Pts',(7.29999999999999,-1.35236351479115,1.04083408558608E-17));
#15044=CARTESIAN_POINT('Ctrl Pts',(8.20044803681595,-1.32637404707459,3.18306896032855E-8));
#15045=CARTESIAN_POINT('Ctrl Pts',(9.10060048441536,-1.28803709316692,1.03188250195688E-8));
#15046=CARTESIAN_POINT('Ctrl Pts',(10.0000000000405,-1.24211782537639,-8.23328475353175E-12));
#15047=CARTESIAN_POINT('Ctrl Pts',(10.0000000000405,1.24211782537639,-8.23320567538283E-12));
#15048=CARTESIAN_POINT('Ctrl Pts',(9.1006004808701,1.28803709334794,1.03184817085883E-8));
#15049=CARTESIAN_POINT('Ctrl Pts',(8.20044803144508,1.32637404722969,3.18291413954212E-8));
#15050=CARTESIAN_POINT('Ctrl Pts',(7.3,1.35236351479115,4.75121773919879E-17));
#15051=CARTESIAN_POINT('',(7.1,1.35793097395724,0.));
#15052=CARTESIAN_POINT('',(7.1,1.42555555555556,0.));
#15053=CARTESIAN_POINT('Ctrl Pts',(7.1000000000396,1.35793097389613,-4.88924676637329E-12));
#15054=CARTESIAN_POINT('Ctrl Pts',(6.53177385320612,1.37316067096195,3.71763852401782E-9));
#15055=CARTESIAN_POINT('Ctrl Pts',(5.96344379069665,1.38333257666104,-3.82408184804385E-8));
#15056=CARTESIAN_POINT('Ctrl Pts',(5.39512359652123,1.38725406840392,-3.97623797275691E-8));
#15057=CARTESIAN_POINT('Ctrl Pts',(4.82973248928002,1.39115534902226,-4.12760989429076E-8));
#15058=CARTESIAN_POINT('Ctrl Pts',(4.26470859812609,1.38886839226708,1.63957607983357E-8));
#15059=CARTESIAN_POINT('Ctrl Pts',(3.70000000036239,1.37924639538501,-6.25376529969227E-12));
#15060=CARTESIAN_POINT('',(3.5,1.37552980833516,0.));
#15061=CARTESIAN_POINT('',(3.5,1.44777777777778,0.));
#15062=CARTESIAN_POINT('Ctrl Pts',(3.50000000097466,1.37552980835479,1.06251812903579E-15));
#15063=CARTESIAN_POINT('Ctrl Pts',(2.69943075695685,1.35940904975719,2.35366119539541E-7));
#15064=CARTESIAN_POINT('Ctrl Pts',(1.89948254587541,1.32827224396921,2.51300192353997E-7));
#15065=CARTESIAN_POINT('Ctrl Pts',(1.10000000028363,1.27885335028943,-5.13283415455519E-11));
#15066=CARTESIAN_POINT('',(0.9,1.266106713614,0.));
#15067=CARTESIAN_POINT('',(0.9,1.34328341716202,0.));
#15068=CARTESIAN_POINT('',(0.292382661757373,1.22257596919059,0.));
#15069=CARTESIAN_POINT('Ctrl Pts',(0.9,1.266106713614,1.20346441145891E-16));
#15070=CARTESIAN_POINT('Ctrl Pts',(0.697432754539207,1.25280566772398,-2.10387859372414E-8));
#15071=CARTESIAN_POINT('Ctrl Pts',(0.494894520889663,1.23831317328004,3.6654767345328E-12));
#15072=CARTESIAN_POINT('Ctrl Pts',(0.292382661757371,1.22257596919059,2.98331735103528E-16));
#15073=CARTESIAN_POINT('Ctrl Pts',(0.292382661757373,1.22257596919059,2.94902990916057E-17));
#15074=CARTESIAN_POINT('Ctrl Pts',(0.284469747869226,1.22196105627757,-8.65621238729993E-13));
#15075=CARTESIAN_POINT('Ctrl Pts',(0.276673396002317,1.22038240716686,-1.19564355630166E-6));
#15076=CARTESIAN_POINT('Ctrl Pts',(0.269153172408756,1.21792571627104,-1.29137975931779E-6));
#15077=CARTESIAN_POINT('Ctrl Pts',(0.264330998492885,1.21635041859408,-1.35276844214688E-6));
#15078=CARTESIAN_POINT('Ctrl Pts',(0.259622238853914,1.21441292414196,-1.0165784587106E-6));
#15079=CARTESIAN_POINT('Ctrl Pts',(0.255072584042237,1.21212521597766,-4.21167369976509E-7));
#15080=CARTESIAN_POINT('Ctrl Pts',(0.247984787860257,1.20856125126747,5.06409032217246E-7));
#15081=CARTESIAN_POINT('Ctrl Pts',(0.241364979299678,1.20419126978451,2.25366520907849E-6));
#15082=CARTESIAN_POINT('Ctrl Pts',(0.235375785094684,1.19908071490398,1.28723124315333E-6));
#15083=CARTESIAN_POINT('Ctrl Pts',(0.235058634311792,1.19881009144014,1.23605486142058E-6));
#15084=CARTESIAN_POINT('Ctrl Pts',(0.234743258170683,1.19853738091759,1.17639378419006E-6));
#15085=CARTESIAN_POINT('Ctrl Pts',(0.234429683218046,1.19826258967301,1.10742116603597E-6));
#15086=CARTESIAN_POINT('Ctrl Pts',(0.23095881299434,1.19522100506769,3.4398325561458E-7));
#15087=CARTESIAN_POINT('Ctrl Pts',(0.227708211416394,1.19192479473749,-1.52348441667556E-6));
#15088=CARTESIAN_POINT('Ctrl Pts',(0.224692430858345,1.18840300965977,-3.42436181452249E-6));
#15089=CARTESIAN_POINT('Ctrl Pts',(0.219522873151367,1.18236607466387,-6.68278702580898E-6));
#15090=CARTESIAN_POINT('Ctrl Pts',(0.21509942609515,1.17573654654733,-9.78259773483875E-6));
#15091=CARTESIAN_POINT('Ctrl Pts',(0.211478909386775,1.16867548752938,-1.04320859863301E-5));
#15092=CARTESIAN_POINT('Ctrl Pts',(0.20968494559888,1.16517673715679,-1.075390701291E-5));
#15093=CARTESIAN_POINT('Ctrl Pts',(0.208088728862602,1.16157146972622,-1.05358292927083E-5));
#15094=CARTESIAN_POINT('Ctrl Pts',(0.206701335101202,1.15787708229469,-9.83193564179307E-6));
#15095=CARTESIAN_POINT('Ctrl Pts',(0.203919119965097,1.15046852899383,-8.42037994342582E-6));
#15096=CARTESIAN_POINT('Ctrl Pts',(0.202003457218558,1.1427818296106,-4.88542801801716E-6));
#15097=CARTESIAN_POINT('Ctrl Pts',(0.201024541128784,1.13496408391561,-2.30807221316776E-6));
#15098=CARTESIAN_POINT('Ctrl Pts',(0.200529226009753,1.13100843574523,-1.00397341389412E-6));
#15099=CARTESIAN_POINT('Ctrl Pts',(0.200274469344113,1.12701892049093,-1.14168925800036E-11));
#15100=CARTESIAN_POINT('Ctrl Pts',(0.200274469199584,1.12301388185427,-1.43114686768087E-17));
#15101=CARTESIAN_POINT('',(-1.73234772679968E-18,1.12356026268968,4.53319947845445E-20));
#15102=CARTESIAN_POINT('',(0.,-1.4,0.));
#15103=CARTESIAN_POINT('',(0.276326924564679,1.42224670711126,-2.77555756156289E-17));
#15104=CARTESIAN_POINT('Ctrl Pts',(0.276326924564681,1.42224670711126,-1.50920942409982E-16));
#15105=CARTESIAN_POINT('Ctrl Pts',(0.258529852003869,1.4208638358667,-3.32972379743633E-13));
#15106=CARTESIAN_POINT('Ctrl Pts',(0.240927013527826,1.41785398988725,-1.99727536601662E-6));
#15107=CARTESIAN_POINT('Ctrl Pts',(0.223720619657732,1.41333325652174,-2.71091968639774E-6));
#15108=CARTESIAN_POINT('Ctrl Pts',(0.206313289378911,1.40875972999491,-3.432897951005E-6));
#15109=CARTESIAN_POINT('Ctrl Pts',(0.18931019325249,1.40263932318529,-2.78724979559428E-6));
#15110=CARTESIAN_POINT('Ctrl Pts',(0.172932985028856,1.39504220432096,-6.31841720307455E-7));
#15111=CARTESIAN_POINT('Ctrl Pts',(0.170060146426803,1.39370954151055,-2.53746782677961E-7));
#15112=CARTESIAN_POINT('Ctrl Pts',(0.167206630967902,1.39233132643846,1.61597591574489E-7));
#15113=CARTESIAN_POINT('Ctrl Pts',(0.164373729059928,1.39090779908693,6.02790108062464E-7));
#15114=CARTESIAN_POINT('Ctrl Pts',(0.148213121449433,1.38278712717586,3.11962244863226E-6));
#15115=CARTESIAN_POINT('Ctrl Pts',(0.132864864406694,1.37326763401578,6.8005293729143E-6));
#15116=CARTESIAN_POINT('Ctrl Pts',(0.118540368157823,1.36244192017091,7.47011412280372E-6));
#15117=CARTESIAN_POINT('Ctrl Pts',(0.1130124780146,1.35826422653222,7.72851001154276E-6));
#15118=CARTESIAN_POINT('Ctrl Pts',(0.107637267132642,1.35389150739715,7.50091387420595E-6));
#15119=CARTESIAN_POINT('Ctrl Pts',(0.102427993107927,1.34932731552598,6.39696583889361E-6));
#15120=CARTESIAN_POINT('Ctrl Pts',(0.0920147884934566,1.34020361352282,
4.19020214765608E-6));
#15121=CARTESIAN_POINT('Ctrl Pts',(0.082263696775192,1.33031540618347,-1.43705507633734E-6));
#15122=CARTESIAN_POINT('Ctrl Pts',(0.0732179607829324,1.31975004019149,
-7.24116446069057E-6));
#15123=CARTESIAN_POINT('Ctrl Pts',(0.0614369648181435,1.30598990677343,
-1.48003270644599E-5));
#15124=CARTESIAN_POINT('Ctrl Pts',(0.0509520748529884,1.29120077200215,
-2.24515165560165E-5));
#15125=CARTESIAN_POINT('Ctrl Pts',(0.0418305631051555,1.27560026299671,
-2.64881615939377E-5));
#15126=CARTESIAN_POINT('Ctrl Pts',(0.0329966685655992,1.26049166530727,
-3.03975241584371E-5));
#15127=CARTESIAN_POINT('Ctrl Pts',(0.0254411283904758,1.24462062939249,
-3.09701348507133E-5));
#15128=CARTESIAN_POINT('Ctrl Pts',(0.0192647836588538,1.2281607987719,-2.81763116144976E-5));
#15129=CARTESIAN_POINT('Ctrl Pts',(0.0129258683931997,1.2112677210496,-2.53089508159798E-5));
#15130=CARTESIAN_POINT('Ctrl Pts',(0.00809110271874438,1.19389182855556,
-1.89493195503086E-5));
#15131=CARTESIAN_POINT('Ctrl Pts',(0.00484442764459327,1.17622983835018,
-1.25518552566888E-5));
#15132=CARTESIAN_POINT('Ctrl Pts',(0.00165723550742335,1.1588914367474,
-6.27160009448058E-6));
#15133=CARTESIAN_POINT('Ctrl Pts',(1.90718451428807E-9,1.14127598190669,
-1.51296892603399E-10));
#15134=CARTESIAN_POINT('Ctrl Pts',(2.41777084464267E-17,1.12356026268968,
-3.46944695195361E-18));
#15135=CARTESIAN_POINT('',(10.5166159648474,1.4155315881283,0.));
#15136=CARTESIAN_POINT('Ctrl Pts',(0.276326924564679,1.42224670711126,0.));
#15137=CARTESIAN_POINT('Ctrl Pts',(3.68975660465893,1.68747752195839,0.));
#15138=CARTESIAN_POINT('Ctrl Pts',(7.10318628475318,1.599994843061,0.));
#15139=CARTESIAN_POINT('Ctrl Pts',(10.5166159648474,1.4155315881283,0.));
#15140=CARTESIAN_POINT('',(10.8,1.11638029377732,-5.56631991785941E-17));
#15141=CARTESIAN_POINT('Ctrl Pts',(10.8,1.11638029377732,2.32452945780892E-16));
#15142=CARTESIAN_POINT('Ctrl Pts',(10.7999999994302,1.13421844616111,-9.29296349749781E-12));
#15143=CARTESIAN_POINT('Ctrl Pts',(10.7983603663884,1.15198349698667,-2.38856955364628E-6));
#15144=CARTESIAN_POINT('Ctrl Pts',(10.7951843826221,1.16946861094468,-3.77014304120448E-6));
#15145=CARTESIAN_POINT('Ctrl Pts',(10.7919669771209,1.18718176881198,-5.16973525142236E-6));
#15146=CARTESIAN_POINT('Ctrl Pts',(10.7871724978816,1.20460918321158,-5.4755482503851E-6));
#15147=CARTESIAN_POINT('Ctrl Pts',(10.7808573412527,1.22152732075962,-4.27334038376583E-6));
#15148=CARTESIAN_POINT('Ctrl Pts',(10.7797421066656,1.22451500471617,-4.06103467663179E-6));
#15149=CARTESIAN_POINT('Ctrl Pts',(10.7785793293545,1.22748675045939,-3.81081650224554E-6));
#15150=CARTESIAN_POINT('Ctrl Pts',(10.7773691713543,1.23044124224994,-3.53261416912234E-6));
#15151=CARTESIAN_POINT('Ctrl Pts',(10.7705159051166,1.24717287467681,-1.95712183132163E-6));
#15152=CARTESIAN_POINT('Ctrl Pts',(10.7622076549587,1.26320448426569,8.50150473021234E-7));
#15153=CARTESIAN_POINT('Ctrl Pts',(10.7525236566209,1.27832128496499,1.09915986206012E-6));
#15154=CARTESIAN_POINT('Ctrl Pts',(10.7482509716548,1.28499098118248,1.20902550183604E-6));
#15155=CARTESIAN_POINT('Ctrl Pts',(10.7437098328292,1.29148238441373,7.76315258636623E-7));
#15156=CARTESIAN_POINT('Ctrl Pts',(10.7389041877712,1.29777551763099,-7.54184826032082E-7));
#15157=CARTESIAN_POINT('Ctrl Pts',(10.7310976851069,1.30799836193882,-3.24039694621926E-6));
#15158=CARTESIAN_POINT('Ctrl Pts',(10.7225935645301,1.31769858917671,-8.57388820182801E-6));
#15159=CARTESIAN_POINT('Ctrl Pts',(10.7134588931078,1.3268364513864,-1.41086939541967E-5));
#15160=CARTESIAN_POINT('Ctrl Pts',(10.7004433550849,1.33985653580309,-2.19949628070403E-5));
#15161=CARTESIAN_POINT('Ctrl Pts',(10.6862650266646,1.35162127070648,-3.0022236679635E-5));
#15162=CARTESIAN_POINT('Ctrl Pts',(10.6711476119081,1.36204513612776,-3.40981369893719E-5));
#15163=CARTESIAN_POINT('Ctrl Pts',(10.6560301971515,1.37246900154903,-3.81740372991087E-5));
#15164=CARTESIAN_POINT('Ctrl Pts',(10.6399721826852,1.38155285075117,-3.83332859284948E-5));
#15165=CARTESIAN_POINT('Ctrl Pts',(10.6231652498763,1.38916602817047,-3.45204725343976E-5));
#15166=CARTESIAN_POINT('Ctrl Pts',(10.6063487480974,1.39678354012646,-3.07054883279539E-5));
#15167=CARTESIAN_POINT('Ctrl Pts',(10.5889271210941,1.40286310406803,-2.29928881382306E-5));
#15168=CARTESIAN_POINT('Ctrl Pts',(10.5711041279812,1.40730078588308,-1.53078138731408E-5));
#15169=CARTESIAN_POINT('Ctrl Pts',(10.5532811348684,1.41173846769814,-7.6227396080509E-6));
#15170=CARTESIAN_POINT('Ctrl Pts',(10.5350552605908,1.41453511891929,-9.16729947674095E-11));
#15171=CARTESIAN_POINT('Ctrl Pts',(10.5166159648474,1.4155315881283,2.48932818802672E-16));
#15172=CARTESIAN_POINT('',(10.8,-1.11638029377732,-1.39157997946485E-17));
#15173=CARTESIAN_POINT('',(10.8,1.4,0.));
#15174=CARTESIAN_POINT('',(10.5166159648474,-1.4155315881283,2.77555756156289E-17));
#15175=CARTESIAN_POINT('Ctrl Pts',(10.5166159648474,-1.4155315881283,-1.94289029309402E-16));
#15176=CARTESIAN_POINT('Ctrl Pts',(10.5344251606169,-1.41456917089032,1.72780596414851E-12));
#15177=CARTESIAN_POINT('Ctrl Pts',(10.5520727686739,-1.41197333457428,-2.53403886306205E-6));
#15178=CARTESIAN_POINT('Ctrl Pts',(10.5693578805681,-1.40785843881911,-4.04156906196095E-6));
#15179=CARTESIAN_POINT('Ctrl Pts',(10.5868701251756,-1.40368947182374,-5.56890876087065E-6));
#15180=CARTESIAN_POINT('Ctrl Pts',(10.604011804524,-1.39796079212135,-5.98742339745246E-6));
#15181=CARTESIAN_POINT('Ctrl Pts',(10.6205627760847,-1.39074087128671,-4.81856832951796E-6));
#15182=CARTESIAN_POINT('Ctrl Pts',(10.6234754753687,-1.38947028374636,-4.61286902618664E-6));
#15183=CARTESIAN_POINT('Ctrl Pts',(10.6263698187278,-1.38815339768352,-4.36721670635639E-6));
#15184=CARTESIAN_POINT('Ctrl Pts',(10.629244514885,-1.38679044403738,-4.09122931699412E-6));
#15185=CARTESIAN_POINT('Ctrl Pts',(10.6455827855986,-1.37904412775797,-2.5226612199239E-6));
#15186=CARTESIAN_POINT('Ctrl Pts',(10.6611432679573,-1.36988219838444,3.58605122725343E-7));
#15187=CARTESIAN_POINT('Ctrl Pts',(10.6757157985124,-1.35939560704671,7.40589063327193E-7));
#15188=CARTESIAN_POINT('Ctrl Pts',(10.6821516119741,-1.35476430808026,9.09288478831296E-7));
#15189=CARTESIAN_POINT('Ctrl Pts',(10.6883944859408,-1.34987400891586,5.44816430868337E-7));
#15190=CARTESIAN_POINT('Ctrl Pts',(10.6944246343503,-1.34472976213865,-9.14752338109426E-7));
#15191=CARTESIAN_POINT('Ctrl Pts',(10.7041966733629,-1.33639335368171,-3.28002794718031E-6));
#15192=CARTESIAN_POINT('Ctrl Pts',(10.7134106653983,-1.3273903805878,-8.47259327327479E-6));
#15193=CARTESIAN_POINT('Ctrl Pts',(10.7220307555455,-1.31778973409553,-1.38734771921913E-5));
#15194=CARTESIAN_POINT('Ctrl Pts',(10.7343338492722,-1.3040871333553,-2.15819326638919E-5));
#15195=CARTESIAN_POINT('Ctrl Pts',(10.7453199276401,-1.28929041974124,-2.94555326738194E-5));
#15196=CARTESIAN_POINT('Ctrl Pts',(10.7549158277293,-1.27362793268665,-3.3443536645081E-5));
#15197=CARTESIAN_POINT('Ctrl Pts',(10.7645117278185,-1.25796544563206,-3.74315406163426E-5));
#15198=CARTESIAN_POINT('Ctrl Pts',(10.7727182208071,-1.24143562566754,-3.75750290962259E-5));
#15199=CARTESIAN_POINT('Ctrl Pts',(10.7794153247677,-1.22423716044977,-3.38265125308188E-5));
#15200=CARTESIAN_POINT('Ctrl Pts',(10.7861166764432,-1.20702778690835,-3.00756184258222E-5));
#15201=CARTESIAN_POINT('Ctrl Pts',(10.7912490477072,-1.18929683429644,-2.25107044755726E-5));
#15202=CARTESIAN_POINT('Ctrl Pts',(10.7947196858669,-1.17125359626911,-1.49815203503087E-5));
#15203=CARTESIAN_POINT('Ctrl Pts',(10.7981903240266,-1.15321035824179,-7.45233622504479E-6));
#15204=CARTESIAN_POINT('Ctrl Pts',(10.7999999985278,-1.13485327409571,-1.17780195603766E-10));
#15205=CARTESIAN_POINT('Ctrl Pts',(10.8,-1.11638029377732,-1.38777878078145E-17));
#15206=CARTESIAN_POINT('',(0.276326924564679,-1.42224670711126,-5.55111512312578E-17));
#15207=CARTESIAN_POINT('Ctrl Pts',(10.5166159648474,-1.4155315881283,0.));
#15208=CARTESIAN_POINT('Ctrl Pts',(7.10318628475318,-1.599994843061,0.));
#15209=CARTESIAN_POINT('Ctrl Pts',(3.68975660465893,-1.68747752195839,0.));
#15210=CARTESIAN_POINT('Ctrl Pts',(0.276326924564679,-1.42224670711126,
0.));
#15211=CARTESIAN_POINT('',(-7.25311916552711E-19,-1.12356026268968,1.39157997946485E-17));
#15212=CARTESIAN_POINT('Ctrl Pts',(1.80411241501588E-16,-1.12356026268968,
-1.53523027623947E-16));
#15213=CARTESIAN_POINT('Ctrl Pts',(7.41078168374529E-10,-1.14141522098415,
-1.3067981184062E-11));
#15214=CARTESIAN_POINT('Ctrl Pts',(0.00163694718329378,-1.15920272117896,
-1.78823819589733E-6));
#15215=CARTESIAN_POINT('Ctrl Pts',(0.00481087395297265,-1.17671209893291,
-2.3181425555783E-6));
#15216=CARTESIAN_POINT('Ctrl Pts',(0.00802138847203439,-1.19442331774104,
-2.85415543927884E-6));
#15217=CARTESIAN_POINT('Ctrl Pts',(0.0128049030182357,-1.21185152247087,
-2.04128886843626E-6));
#15218=CARTESIAN_POINT('Ctrl Pts',(0.0191087770915565,-1.22877027194193,
1.71240493184593E-7));
#15219=CARTESIAN_POINT('Ctrl Pts',(0.0202201941454154,-1.23175316571065,
5.613248819379E-7));
#15220=CARTESIAN_POINT('Ctrl Pts',(0.0213789882593307,-1.23472016785247,
9.85829603970989E-7));
#15221=CARTESIAN_POINT('Ctrl Pts',(0.0225850188675993,-1.23766995297306,
1.43287414332239E-6));
#15222=CARTESIAN_POINT('Ctrl Pts',(0.0294291562303479,-1.25440977235863,
3.96981990042924E-6));
#15223=CARTESIAN_POINT('Ctrl Pts',(0.0377300686697735,-1.27044838970616,
7.55798501181421E-6));
#15224=CARTESIAN_POINT('Ctrl Pts',(0.0474121614036163,-1.28556782977674,
8.05058320302158E-6));
#15225=CARTESIAN_POINT('Ctrl Pts',(0.0511425121829324,-1.29139310088294,
8.24037316857697E-6));
#15226=CARTESIAN_POINT('Ctrl Pts',(0.0550784035723718,-1.29708174651376,
7.93435480917585E-6));
#15227=CARTESIAN_POINT('Ctrl Pts',(0.0592173503759339,-1.30262033374061,
6.74858081742264E-6));
#15228=CARTESIAN_POINT('Ctrl Pts',(0.0675201807396794,-1.31373087764993,
4.36988865960166E-6));
#15229=CARTESIAN_POINT('Ctrl Pts',(0.0766394565597649,-1.32423847988766,
-1.46587651676554E-6));
#15230=CARTESIAN_POINT('Ctrl Pts',(0.0864911062490747,-1.33409287340636,
-7.46705500292641E-6));
#15231=CARTESIAN_POINT('Ctrl Pts',(0.0992988409846585,-1.34690417528452,
-1.52689465211603E-5));
#15232=CARTESIAN_POINT('Ctrl Pts',(0.113232871116931,-1.35850278376499,
-2.31308069859054E-5));
#15233=CARTESIAN_POINT('Ctrl Pts',(0.128081622025101,-1.36880445085772,
-2.72849174168177E-5));
#15234=CARTESIAN_POINT('Ctrl Pts',(0.142447925282442,-1.37877140864598,
-3.13040575171566E-5));
#15235=CARTESIAN_POINT('Ctrl Pts',(0.157671864768995,-1.38752483454192,
-3.1899138628041E-5));
#15236=CARTESIAN_POINT('Ctrl Pts',(0.173588691395025,-1.39495074934422,
-2.90326641197332E-5));
#15237=CARTESIAN_POINT('Ctrl Pts',(0.189936400238013,-1.40257769006131,
-2.60885916756054E-5));
#15238=CARTESIAN_POINT('Ctrl Pts',(0.206881864105471,-1.40874232120582,
-1.95409011442111E-5));
#15239=CARTESIAN_POINT('Ctrl Pts',(0.22423558959196,-1.41334558507228,-1.29462590315495E-5));
#15240=CARTESIAN_POINT('Ctrl Pts',(0.241260467995769,-1.4178616186841,-6.47658310103417E-6));
#15241=CARTESIAN_POINT('Ctrl Pts',(0.258679581942429,-1.42087546890512,
-1.12101563992788E-10));
#15242=CARTESIAN_POINT('Ctrl Pts',(0.27632692456468,-1.42224670711126,1.05818132034585E-16));
#15243=CARTESIAN_POINT('',(0.,-1.4,0.));
#15244=CARTESIAN_POINT('',(0.292382661757373,-1.22257596919059,0.));
#15245=CARTESIAN_POINT('Ctrl Pts',(0.200274469199584,-1.12301388185427,
-2.68882138776405E-17));
#15246=CARTESIAN_POINT('Ctrl Pts',(0.200274469314753,-1.13095194822878,
-2.85686379674833E-12));
#15247=CARTESIAN_POINT('Ctrl Pts',(0.201244085522878,-1.13884856843413,
-1.08105759021766E-6));
#15248=CARTESIAN_POINT('Ctrl Pts',(0.203110344361254,-1.14653799330522,
-1.10782444979703E-6));
#15249=CARTESIAN_POINT('Ctrl Pts',(0.204308287281872,-1.15147379958167,
-1.12500597321754E-6));
#15250=CARTESIAN_POINT('Ctrl Pts',(0.205876831658669,-1.15632444796435,
-7.573778542164E-7));
#15251=CARTESIAN_POINT('Ctrl Pts',(0.207807574899602,-1.16104329283393,
-1.57887042599725E-7));
#15252=CARTESIAN_POINT('Ctrl Pts',(0.21096922807971,-1.1687705506961,8.23798139982571E-7));
#15253=CARTESIAN_POINT('Ctrl Pts',(0.215060220496011,-1.17605061753432,
2.67511715935828E-6));
#15254=CARTESIAN_POINT('Ctrl Pts',(0.220020901709485,-1.18268777995331,
1.20301732358232E-6));
#15255=CARTESIAN_POINT('Ctrl Pts',(0.222788929945646,-1.18639127392786,
3.81595076007225E-7));
#15256=CARTESIAN_POINT('Ctrl Pts',(0.225828882930032,-1.18989419630164,
-1.55522758636672E-6));
#15257=CARTESIAN_POINT('Ctrl Pts',(0.229112809647272,-1.19317965616817,
-3.52099818518546E-6));
#15258=CARTESIAN_POINT('Ctrl Pts',(0.234731790749985,-1.1988012605745,-6.88454091865859E-6));
#15259=CARTESIAN_POINT('Ctrl Pts',(0.240999377733319,-1.20372479786492,
-1.00686973618824E-5));
#15260=CARTESIAN_POINT('Ctrl Pts',(0.247759525934523,-1.2078808899968,-1.07387199666626E-5));
#15261=CARTESIAN_POINT('Ctrl Pts',(0.251104201987095,-1.20993717358883,
-1.10702228411842E-5));
#15262=CARTESIAN_POINT('Ctrl Pts',(0.254570062984725,-1.21180502729412,
-1.08478245319173E-5));
#15263=CARTESIAN_POINT('Ctrl Pts',(0.258140701417296,-1.21347208138814,
-1.01264154182862E-5));
#15264=CARTESIAN_POINT('Ctrl Pts',(0.265309933881728,-1.21681924144269,
-8.67794906268977E-6));
#15265=CARTESIAN_POINT('Ctrl Pts',(0.27282354441991,-1.21932394229889,-5.03816435877804E-6));
#15266=CARTESIAN_POINT('Ctrl Pts',(0.280540402387729,-1.22090470300999,
-2.38011023443526E-6));
#15267=CARTESIAN_POINT('Ctrl Pts',(0.284441227387562,-1.22170376798259,
-1.03647996128718E-6));
#15268=CARTESIAN_POINT('Ctrl Pts',(0.288394358015454,-1.22226603782358,
-8.41267709508591E-12));
#15269=CARTESIAN_POINT('Ctrl Pts',(0.292382661757373,-1.22257596919059,
3.10081821330854E-17));
#15270=CARTESIAN_POINT('',(0.9,-1.266106713614,0.));
#15271=CARTESIAN_POINT('Ctrl Pts',(0.29238266175737,-1.22257596919059,3.4274341177698E-16));
#15272=CARTESIAN_POINT('Ctrl Pts',(0.494894519961671,-1.23831317320793,
3.6654050078524E-12));
#15273=CARTESIAN_POINT('Ctrl Pts',(0.697432753591781,-1.25280566766171,
-2.10377631034678E-8));
#15274=CARTESIAN_POINT('Ctrl Pts',(0.900000000000002,-1.266106713614,4.80511808774455E-17));
#15275=CARTESIAN_POINT('',(0.9,1.34328341716202,0.));
#15276=CARTESIAN_POINT('',(3.5,-1.37552980833516,0.));
#15277=CARTESIAN_POINT('Ctrl Pts',(1.10000000028363,-1.27885335028943,-5.13283219638443E-11));
#15278=CARTESIAN_POINT('Ctrl Pts',(1.8994825293422,-1.32827224294784,2.51289069808066E-7));
#15279=CARTESIAN_POINT('Ctrl Pts',(2.69943073922525,-1.35940904940056,2.35357980118634E-7));
#15280=CARTESIAN_POINT('Ctrl Pts',(3.50000000097418,-1.37552980835478,8.59034485311056E-16));
#15281=CARTESIAN_POINT('',(3.5,1.44777777777778,0.));
#15282=CARTESIAN_POINT('',(7.1,-1.35793097395724,0.));
#15283=CARTESIAN_POINT('Ctrl Pts',(3.700000000362,-1.379246395385,-6.25385501848083E-12));
#15284=CARTESIAN_POINT('Ctrl Pts',(4.26467016042339,-1.38886773733237,1.63880713394601E-8));
#15285=CARTESIAN_POINT('Ctrl Pts',(4.82965558050887,-1.39115503781354,-4.12727732537403E-8));
#15286=CARTESIAN_POINT('Ctrl Pts',(5.39500817395676,-1.38725486475042,-3.97626883737645E-8));
#15287=CARTESIAN_POINT('Ctrl Pts',(5.96336684492344,-1.38333395379258,-3.82445741104923E-8));
#15288=CARTESIAN_POINT('Ctrl Pts',(6.53173538886785,-1.37316170188981,3.71969681223073E-9));
#15289=CARTESIAN_POINT('Ctrl Pts',(7.1000000000396,-1.35793097389613,-4.88946831112289E-12));
#15290=CARTESIAN_POINT('',(7.1,1.42555555555556,0.));
#15291=CARTESIAN_POINT('',(10.2,-1.23178301601145,0.));
#15292=CARTESIAN_POINT('',(10.5052647440597,-1.21555035534119,0.));
#15293=CARTESIAN_POINT('Ctrl Pts',(10.2,-1.23178301601145,-4.56855690431079E-17));
#15294=CARTESIAN_POINT('Ctrl Pts',(10.3017652114452,-1.22646242153193,-6.28718440835499E-11));
#15295=CARTESIAN_POINT('Ctrl Pts',(10.4035203469111,-1.22104923788321,1.43982679105611E-13));
#15296=CARTESIAN_POINT('Ctrl Pts',(10.5052647440597,-1.21555035534119,6.44897004721534E-17));
#15297=CARTESIAN_POINT('',(10.5997255308004,-1.11583328740478,1.38777878078145E-17));
#15298=CARTESIAN_POINT('Ctrl Pts',(10.5052647440597,-1.21555035534119,-1.86482773667507E-17));
#15299=CARTESIAN_POINT('Ctrl Pts',(10.5131888530666,-1.21512208850275,-5.60416335832109E-13));
#15300=CARTESIAN_POINT('Ctrl Pts',(10.5210180054001,-1.21372544600509,-1.35972994235015E-6));
#15301=CARTESIAN_POINT('Ctrl Pts',(10.5285917824072,-1.2114444991589,-1.66070161277884E-6));
#15302=CARTESIAN_POINT('Ctrl Pts',(10.5334522234388,-1.20998071066451,-1.8538489757029E-6));
#15303=CARTESIAN_POINT('Ctrl Pts',(10.538207639053,-1.20815156029678,-1.66445033219183E-6));
#15304=CARTESIAN_POINT('Ctrl Pts',(10.542812250732,-1.20596855068549,-1.19054254011085E-6));
#15305=CARTESIAN_POINT('Ctrl Pts',(10.5499808226381,-1.20256998801374,-4.52751316616249E-7));
#15306=CARTESIAN_POINT('Ctrl Pts',(10.5567010840309,-1.19835579238971,1.16775294480959E-6));
#15307=CARTESIAN_POINT('Ctrl Pts',(10.5628099082467,-1.1933896765605,3.12218506849373E-7));
#15308=CARTESIAN_POINT('Ctrl Pts',(10.563392699667,-1.1929159013142,2.30599178383296E-7));
#15309=CARTESIAN_POINT('Ctrl Pts',(10.563969906567,-1.19243524850296,1.23643260424227E-7));
#15310=CARTESIAN_POINT('Ctrl Pts',(10.5645413730323,-1.19194775268147,-1.33988689923433E-8));
#15311=CARTESIAN_POINT('Ctrl Pts',(10.5677990734116,-1.18916873515523,-7.94620907596477E-7));
#15312=CARTESIAN_POINT('Ctrl Pts',(10.5708705204042,-1.18616755700159,-2.52696578471864E-6));
#15313=CARTESIAN_POINT('Ctrl Pts',(10.5737438185805,-1.18296717200411,-4.3349897000341E-6));
#15314=CARTESIAN_POINT('Ctrl Pts',(10.579054042416,-1.17705244973962,-7.67644996655303E-6));
#15315=CARTESIAN_POINT('Ctrl Pts',(10.5836289246435,-1.17052745137283,-1.0999028846932E-5));
#15316=CARTESIAN_POINT('Ctrl Pts',(10.5874112735695,-1.16355342251842,-1.18035167459916E-5));
#15317=CARTESIAN_POINT('Ctrl Pts',(10.5894705469099,-1.15975646143,-1.22415145393192E-5));
#15318=CARTESIAN_POINT('Ctrl Pts',(10.5912942421259,-1.15582570378367,-1.20038889321768E-5));
#15319=CARTESIAN_POINT('Ctrl Pts',(10.5928674986933,-1.15178403025788,-1.11465830745351E-5));
#15320=CARTESIAN_POINT('Ctrl Pts',(10.5957384082276,-1.14440870489779,-9.58215448007377E-6));
#15321=CARTESIAN_POINT('Ctrl Pts',(10.5977463817932,-1.13674651935037,-5.80208140981121E-6));
#15322=CARTESIAN_POINT('Ctrl Pts',(10.5988207707371,-1.12894377506163,-2.8960211281105E-6));
#15323=CARTESIAN_POINT('Ctrl Pts',(10.5994175893465,-1.12460938291963,-1.28171667533415E-6));
#15324=CARTESIAN_POINT('Ctrl Pts',(10.5997255306822,-1.12023121224821,-9.4020583932734E-12));
#15325=CARTESIAN_POINT('Ctrl Pts',(10.5997255308004,-1.11583328740478,-9.97465998686664E-18));
#15326=CARTESIAN_POINT('',(10.5997255308004,1.11583328740478,0.));
#15327=CARTESIAN_POINT('',(10.5997255308004,0.7,0.));
#15328=CARTESIAN_POINT('',(10.5052647440597,1.21555035534119,0.));
#15329=CARTESIAN_POINT('Ctrl Pts',(10.5997255308004,1.11583328740478,8.8037216405823E-17));
#15330=CARTESIAN_POINT('Ctrl Pts',(10.5997255307124,1.12376989384288,-2.22024716398596E-12));
#15331=CARTESIAN_POINT('Ctrl Pts',(10.5987536115518,1.13166401228391,-1.27532141444775E-6));
#15332=CARTESIAN_POINT('Ctrl Pts',(10.5968849989732,1.13935090273995,-1.5236651967046E-6));
#15333=CARTESIAN_POINT('Ctrl Pts',(10.5956849616024,1.14428748291596,-1.68315348385219E-6));
#15334=CARTESIAN_POINT('Ctrl Pts',(10.5941139374364,1.14913880701507,-1.46899737395989E-6));
#15335=CARTESIAN_POINT('Ctrl Pts',(10.5921809408638,1.1538584293407,-9.90118991603547E-7));
#15336=CARTESIAN_POINT('Ctrl Pts',(10.5891742477341,1.16119959911942,-2.45244239835432E-7));
#15337=CARTESIAN_POINT('Ctrl Pts',(10.5853292249979,1.16813727090899,1.33309554558619E-6));
#15338=CARTESIAN_POINT('Ctrl Pts',(10.5807005079991,1.17450509276749,4.08358240744415E-7));
#15339=CARTESIAN_POINT('Ctrl Pts',(10.5802604812716,1.17511044665166,3.20448539159982E-7));
#15340=CARTESIAN_POINT('Ctrl Pts',(10.5798133373602,1.17571063303672,2.07176952714776E-7));
#15341=CARTESIAN_POINT('Ctrl Pts',(10.5793591019426,1.17630549598644,6.38823567561716E-8));
#15342=CARTESIAN_POINT('Ctrl Pts',(10.5767566952267,1.17971358631841,-7.57081408668461E-7));
#15343=CARTESIAN_POINT('Ctrl Pts',(10.5739217504488,1.18294722379721,-2.53660858190298E-6));
#15344=CARTESIAN_POINT('Ctrl Pts',(10.570876618072,1.18599321478588,-4.38998728286835E-6));
#15345=CARTESIAN_POINT('Ctrl Pts',(10.5652565693637,1.19161484813492,-7.81055403847458E-6));
#15346=CARTESIAN_POINT('Ctrl Pts',(10.5589874561388,1.19653507038546,-1.11999964534866E-5));
#15347=CARTESIAN_POINT('Ctrl Pts',(10.5522271124844,1.20068789486255,-1.20263298844839E-5));
#15348=CARTESIAN_POINT('Ctrl Pts',(10.5485500617744,1.20294667739977,-1.24757848359648E-5));
#15349=CARTESIAN_POINT('Ctrl Pts',(10.5447269560479,1.20497781184918,-1.22374322375965E-5));
#15350=CARTESIAN_POINT('Ctrl Pts',(10.5407797717187,1.20676523914267,-1.13674773191707E-5));
#15351=CARTESIAN_POINT('Ctrl Pts',(10.5335711832013,1.210029547771,-9.77871264224002E-6));
#15352=CARTESIAN_POINT('Ctrl Pts',(10.5260296312848,1.21244761587922,-5.9245235663186E-6));
#15353=CARTESIAN_POINT('Ctrl Pts',(10.5182973307397,1.21394093281975,-2.95733858081469E-6));
#15354=CARTESIAN_POINT('Ctrl Pts',(10.514004731837,1.21476995008607,-1.31010113336685E-6));
#15355=CARTESIAN_POINT('Ctrl Pts',(10.5096528988527,1.21531319279956,-7.28166367327128E-12));
#15356=CARTESIAN_POINT('Ctrl Pts',(10.5052647440597,1.21555035534119,-3.31765864780564E-17));
#15357=CARTESIAN_POINT('',(10.2,1.23178301601145,0.));
#15358=CARTESIAN_POINT('Ctrl Pts',(10.5052647440597,1.21555035534119,1.20285454773689E-16));
#15359=CARTESIAN_POINT('Ctrl Pts',(10.4035203468995,1.22104923788384,1.44021921739714E-13));
#15360=CARTESIAN_POINT('Ctrl Pts',(10.3017652114309,1.22646242153268,-6.28696045710378E-11));
#15361=CARTESIAN_POINT('Ctrl Pts',(10.2,1.23178301601145,1.23125603768043E-16));
#15362=CARTESIAN_POINT('',(10.2,-1.30754691548544,0.));
#15363=CARTESIAN_POINT('Origin',(8.8,0.,0.));
#15364=CARTESIAN_POINT('',(8.4,-4.89858719658942E-17,0.));
#15365=CARTESIAN_POINT('Origin',(2.,0.,0.));
#15366=CARTESIAN_POINT('',(1.6,-4.89858719658941E-17,0.7));
#15367=CARTESIAN_POINT('Origin',(2.,0.,0.7));
#15368=CARTESIAN_POINT('',(1.6,-4.89858719658941E-17,0.));
#15369=CARTESIAN_POINT('Origin',(10.2,-1.30754691548544,0.));
#15370=CARTESIAN_POINT('',(10.1999999975107,-1.19856231453552,0.605472757505173));
#15371=CARTESIAN_POINT('Ctrl Pts',(10.2,-1.23178301601145,0.));
#15372=CARTESIAN_POINT('Ctrl Pts',(10.2,-1.22625045235593,0.100869147801815));
#15373=CARTESIAN_POINT('Ctrl Pts',(10.2,-1.22071692450357,0.201739022585575));
#15374=CARTESIAN_POINT('Ctrl Pts',(10.2,-1.2096433936729,0.403562754186249));
#15375=CARTESIAN_POINT('Ctrl Pts',(10.1999999975107,-1.20410330368611,0.50451817268257));
#15376=CARTESIAN_POINT('Ctrl Pts',(10.1999999975107,-1.19856231453552,0.605472757505173));
#15377=CARTESIAN_POINT('',(10.1999999975107,1.19856231453552,0.605472757505173));
#15378=CARTESIAN_POINT('Ctrl Pts',(10.1999999975107,1.19856231453552,0.605472757505173));
#15379=CARTESIAN_POINT('Ctrl Pts',(10.1999999975107,1.20410418062036,0.504502195294633));
#15380=CARTESIAN_POINT('Ctrl Pts',(10.2,1.20964514726505,0.403530798997214));
#15381=CARTESIAN_POINT('Ctrl Pts',(10.2,1.22071867750565,0.201707067365009));
#15382=CARTESIAN_POINT('Ctrl Pts',(10.2,1.22625132869937,0.100853170395858));
#15383=CARTESIAN_POINT('Ctrl Pts',(10.2,1.23178301601145,0.));
#15384=CARTESIAN_POINT('',(10.1999999980542,1.09857320530976,0.7));
#15385=CARTESIAN_POINT('Ctrl Pts',(10.1999999999973,1.09857320510493,0.7));
#15386=CARTESIAN_POINT('Ctrl Pts',(10.2000000008642,1.10649088744708,0.699999999248278));
#15387=CARTESIAN_POINT('Ctrl Pts',(10.1999989363772,1.11434529358656,0.699006164779054));
#15388=CARTESIAN_POINT('Ctrl Pts',(10.1999980093114,1.12199598895487,0.697118997523365));
#15389=CARTESIAN_POINT('Ctrl Pts',(10.1999974900707,1.12628106973794,0.696062013320951));
#15390=CARTESIAN_POINT('Ctrl Pts',(10.1999970168623,1.13050229860485,0.694723760583242));
#15391=CARTESIAN_POINT('Ctrl Pts',(10.199996713894,1.13463332887353,0.693115046692397));
#15392=CARTESIAN_POINT('Ctrl Pts',(10.1999961690675,1.14206214329588,0.690222103243312));
#15393=CARTESIAN_POINT('Ctrl Pts',(10.1999962772589,1.14911941279843,0.686488866209959));
#15394=CARTESIAN_POINT('Ctrl Pts',(10.1999969599022,1.15565885618684,0.681996408643444));
#15395=CARTESIAN_POINT('Ctrl Pts',(10.1999973343062,1.15924549304116,0.679532465931891));
#15396=CARTESIAN_POINT('Ctrl Pts',(10.1999978674396,1.16267609380848,0.676839263748528));
#15397=CARTESIAN_POINT('Ctrl Pts',(10.1999983417863,1.16592263776853,0.673924718551186));
#15398=CARTESIAN_POINT('Ctrl Pts',(10.199998806773,1.16910511991263,0.671067684066867));
#15399=CARTESIAN_POINT('Ctrl Pts',(10.1999992207276,1.17209141256199,0.668015240668471));
#15400=CARTESIAN_POINT('Ctrl Pts',(10.1999992206607,1.17485880184773,0.664778864469812));
#15401=CARTESIAN_POINT('Ctrl Pts',(10.1999992205369,1.17997899231675,0.658790960038769));
#15402=CARTESIAN_POINT('Ctrl Pts',(10.1999979581638,1.18435276586188,0.652174799271591));
#15403=CARTESIAN_POINT('Ctrl Pts',(10.1999975326045,1.18791964688485,0.645095405674036));
#15404=CARTESIAN_POINT('Ctrl Pts',(10.1999974898604,1.18827791229431,0.644384335742179));
#15405=CARTESIAN_POINT('Ctrl Pts',(10.1999974535047,1.18862799840101,0.643668573506599));
#15406=CARTESIAN_POINT('Ctrl Pts',(10.1999974242393,1.18896981696374,0.64294827577739));
#15407=CARTESIAN_POINT('Ctrl Pts',(10.1999971329942,1.1923715530028,0.635779961907205));
#15408=CARTESIAN_POINT('Ctrl Pts',(10.1999977790614,1.19491900203126,0.628247233077589));
#15409=CARTESIAN_POINT('Ctrl Pts',(10.1999987199397,1.19655829940385,0.620518158911201));
#15410=CARTESIAN_POINT('Ctrl Pts',(10.1999993222661,1.19760773597399,0.615570201805241));
#15411=CARTESIAN_POINT('Ctrl Pts',(10.2,1.19828413277105,0.610541112135461));
#15412=CARTESIAN_POINT('Ctrl Pts',(10.2,1.19856231427281,0.60547275750556));
#15413=CARTESIAN_POINT('',(10.2,-1.09857320510402,0.7));
#15414=CARTESIAN_POINT('',(10.2,-0.653773457742722,0.7));
#15415=CARTESIAN_POINT('Ctrl Pts',(10.2,-1.19856231427281,0.60547275750556));
#15416=CARTESIAN_POINT('Ctrl Pts',(10.2,-1.19812809376428,0.613384079828744));
#15417=CARTESIAN_POINT('Ctrl Pts',(10.1999984889428,-1.1967261327477,0.621202329970501));
#15418=CARTESIAN_POINT('Ctrl Pts',(10.1999978161146,-1.19444079525024,0.628767398200536));
#15419=CARTESIAN_POINT('Ctrl Pts',(10.1999974438306,-1.19317629038787,0.632953241898348));
#15420=CARTESIAN_POINT('Ctrl Pts',(10.1999972759003,-1.19164034846853,0.637061602680377));
#15421=CARTESIAN_POINT('Ctrl Pts',(10.1999973648938,-1.18984073583679,0.641063423920242));
#15422=CARTESIAN_POINT('Ctrl Pts',(10.1999975257516,-1.18658789218766,0.648296813248274));
#15423=CARTESIAN_POINT('Ctrl Pts',(10.1999986492083,-1.18251199594868,0.655103972585077));
#15424=CARTESIAN_POINT('Ctrl Pts',(10.1999990866637,-1.1776776067306,0.66132208754656));
#15425=CARTESIAN_POINT('Ctrl Pts',(10.1999991692372,-1.17676507450965,0.662495809810115));
#15426=CARTESIAN_POINT('Ctrl Pts',(10.1999992204458,-1.17582538639523,0.663648473741297));
#15427=CARTESIAN_POINT('Ctrl Pts',(10.1999992199672,-1.17485880188435,0.664778864469789));
#15428=CARTESIAN_POINT('Ctrl Pts',(10.1999992190419,-1.17299032792757,0.666963987046661));
#15429=CARTESIAN_POINT('Ctrl Pts',(10.1999990265713,-1.17102137903347,0.669065925022507));
#15430=CARTESIAN_POINT('Ctrl Pts',(10.1999987631451,-1.16895889720817,0.671081139337088));
#15431=CARTESIAN_POINT('Ctrl Pts',(10.1999980371048,-1.16327440276409,0.676635357771578));
#15432=CARTESIAN_POINT('Ctrl Pts',(10.1999968952367,-1.15694629605269,0.681471105251756));
#15433=CARTESIAN_POINT('Ctrl Pts',(10.1999965193249,-1.15013861030111,0.685534582868085));
#15434=CARTESIAN_POINT('Ctrl Pts',(10.1999962798276,-1.14580136285465,0.688123466749966));
#15435=CARTESIAN_POINT('Ctrl Pts',(10.1999963003895,-1.14126848503633,0.690398200126003));
#15436=CARTESIAN_POINT('Ctrl Pts',(10.1999965837416,-1.13657664085124,0.692335536714198));
#15437=CARTESIAN_POINT('Ctrl Pts',(10.199997026059,-1.12925259320479,0.695359751696499));
#15438=CARTESIAN_POINT('Ctrl Pts',(10.1999981114625,-1.12162598460505,0.697529439192009));
#15439=CARTESIAN_POINT('Ctrl Pts',(10.1999989867727,-1.11384404680861,0.698775198878229));
#15440=CARTESIAN_POINT('Ctrl Pts',(10.1999995533653,-1.10880676031141,0.699581585232154));
#15441=CARTESIAN_POINT('Ctrl Pts',(10.200000000559,-1.10370379302489,0.699999999512891));
#15442=CARTESIAN_POINT('Ctrl Pts',(10.1999999999973,-1.09857320510493,0.7));
#15443=CARTESIAN_POINT('Ctrl Pts',(10.0273290644374,-1.24073895154929,-0.000342977371441382));
#15444=CARTESIAN_POINT('Ctrl Pts',(10.0182194939277,-1.2301570933055,0.201590462913323));
#15445=CARTESIAN_POINT('Ctrl Pts',(10.0091098064739,-1.21957524432673,0.403523898419685));
#15446=CARTESIAN_POINT('Ctrl Pts',(10.,-1.20899340483173,0.605457329065658));
#15447=CARTESIAN_POINT('Ctrl Pts',(9.11786336174441,-1.287320026752,-0.000205293215301774));
#15448=CARTESIAN_POINT('Ctrl Pts',(9.11054075262461,-1.27673792859995,0.201728409731728));
#15449=CARTESIAN_POINT('Ctrl Pts',(9.10321803982027,-1.2661558351744,0.403662109352091));
#15450=CARTESIAN_POINT('Ctrl Pts',(9.09589522044064,-1.25557375159922,0.605595805683776));
#15451=CARTESIAN_POINT('Ctrl Pts',(8.20875307681921,-1.32613868191631,-8.19769783003664E-5));
#15452=CARTESIAN_POINT('Ctrl Pts',(8.20321812688803,-1.31555630757271,0.201851960079368));
#15453=CARTESIAN_POINT('Ctrl Pts',(8.19768309032111,-1.30497393555236,0.403785895133155));
#15454=CARTESIAN_POINT('Ctrl Pts',(8.19214796413157,-1.29439157095064,0.605719828258773));
#15455=CARTESIAN_POINT('Ctrl Pts',(7.29999999999999,-1.35236351479115,1.04083408558608E-17));
#15456=CARTESIAN_POINT('Ctrl Pts',(7.29625341766944,-1.34178092325774,0.201934092022114));
#15457=CARTESIAN_POINT('Ctrl Pts',(7.2925067690755,-1.33119833465137,0.403868182971915));
#15458=CARTESIAN_POINT('Ctrl Pts',(7.28876005303739,-1.32061574904145,0.605802272831199));
#15459=CARTESIAN_POINT('Ctrl Pts',(7.29999999953094,-1.32031613471704,0.605285370449856));
#15460=CARTESIAN_POINT('Ctrl Pts',(8.20058408060299,-1.29406305600824,0.605326635812744));
#15461=CARTESIAN_POINT('Ctrl Pts',(9.10058974048747,-1.25534320916473,0.605388449123016));
#15462=CARTESIAN_POINT('Ctrl Pts',(9.99999999968202,-1.20899340489109,0.605457329065633));
#15463=CARTESIAN_POINT('Ctrl Pts',(10.5052670937641,-1.21555282972197,-4.72190879230918E-5));
#15464=CARTESIAN_POINT('Ctrl Pts',(10.4952228315222,-1.20497561405085,0.201799837144789));
#15465=CARTESIAN_POINT('Ctrl Pts',(10.4851784461209,-1.19439840869387,0.403646887802288));
#15466=CARTESIAN_POINT('Ctrl Pts',(10.4751339353761,-1.18382121389426,0.605493932788863));
#15467=CARTESIAN_POINT('Ctrl Pts',(10.4035069533234,-1.22105168617584,-3.13467776074076E-5));
#15468=CARTESIAN_POINT('Ctrl Pts',(10.3936624949941,-1.21047444506522,0.201815739766394));
#15469=CARTESIAN_POINT('Ctrl Pts',(10.3838179147697,-1.19989721405033,0.403662820908308));
#15470=CARTESIAN_POINT('Ctrl Pts',(10.3739732104882,-1.18931999337004,0.605509896555428));
#15471=CARTESIAN_POINT('Ctrl Pts',(10.3017512542637,-1.22646400658821,-1.55943981238903E-5));
#15472=CARTESIAN_POINT('Ctrl Pts',(10.2921066085356,-1.21588673949083,0.201831522212972));
#15473=CARTESIAN_POINT('Ctrl Pts',(10.2824618422276,-1.20530948226626,0.403678633593635));
#15474=CARTESIAN_POINT('Ctrl Pts',(10.2728169532007,-1.19473223514815,0.605525739654126));
#15475=CARTESIAN_POINT('Ctrl Pts',(10.2,-1.23178301601145,-4.5102810375397E-17));
#15476=CARTESIAN_POINT('Ctrl Pts',(10.1905551755811,-1.22120572247414,0.20184714636246));
#15477=CARTESIAN_POINT('Ctrl Pts',(10.1811102319487,-1.21062843858304,0.403694287664275));
#15478=CARTESIAN_POINT('Ctrl Pts',(10.1716651669877,-1.20005116456574,0.605541423818621));
#15479=CARTESIAN_POINT('',(10.4735630903435,-1.18390659316268,0.605494180667944));
#15480=CARTESIAN_POINT('Ctrl Pts',(10.1999999975038,-1.19856231440453,0.605472757505366));
#15481=CARTESIAN_POINT('Ctrl Pts',(10.2911933328565,-1.19375025772558,0.605479840815741));
#15482=CARTESIAN_POINT('Ctrl Pts',(10.3823809652617,-1.18886335120032,0.605486986548286));
#15483=CARTESIAN_POINT('Ctrl Pts',(10.4735630903435,-1.18390659316268,0.605494180667944));
#15484=CARTESIAN_POINT('Ctrl Pts',(10.4735630903435,-1.18390659316268,0.605494180667945));
#15485=CARTESIAN_POINT('Ctrl Pts',(10.4841302498201,-1.19445434834508,0.403662775875149));
#15486=CARTESIAN_POINT('Ctrl Pts',(10.4946974680575,-1.20500226999407,0.201831382381129));
#15487=CARTESIAN_POINT('Ctrl Pts',(10.5052647440597,-1.21555035534119,-6.86299975183324E-17));
#15488=CARTESIAN_POINT('Ctrl Pts',(10.,-1.10900986674273,0.7));
#15489=CARTESIAN_POINT('Ctrl Pts',(9.09944331332257,-1.15544418981837,0.7));
#15490=CARTESIAN_POINT('Ctrl Pts',(8.1984670949788,-1.19422430779862,0.7));
#15491=CARTESIAN_POINT('Ctrl Pts',(7.29709043526679,-1.22049830417059,0.7));
#15492=CARTESIAN_POINT('Ctrl Pts',(10.0014871213396,-1.13785139984992,0.7));
#15493=CARTESIAN_POINT('Ctrl Pts',(9.10076698492608,-1.18430758604571,0.700000491839571));
#15494=CARTESIAN_POINT('Ctrl Pts',(8.19957769811723,-1.22310890030201,0.699999704549177));
#15495=CARTESIAN_POINT('Ctrl Pts',(7.29793284700475,-1.24939875264889,0.7));
#15496=CARTESIAN_POINT('Ctrl Pts',(10.0040646682326,-1.18784086746588,0.676686753673613));
#15497=CARTESIAN_POINT('Ctrl Pts',(9.10306300621911,-1.23433322993607,0.676664155483858));
#15498=CARTESIAN_POINT('Ctrl Pts',(8.20149954052229,-1.27317186922949,0.676644146017133));
#15499=CARTESIAN_POINT('Ctrl Pts',(7.29939288958795,-1.29948813715084,0.676630595533454));
#15500=CARTESIAN_POINT('Ctrl Pts',(10.0050807923581,-1.20754778500352,0.627085325222079));
#15501=CARTESIAN_POINT('Ctrl Pts',(9.10396596140607,-1.25402923300358,0.627026849623412));
#15502=CARTESIAN_POINT('Ctrl Pts',(8.20225661204673,-1.29285896783792,0.626974637782525));
#15503=CARTESIAN_POINT('Ctrl Pts',(7.29996660609514,-1.31917051289423,0.626939603849942));
#15504=CARTESIAN_POINT('Ctrl Pts',(10.0051416645797,-1.20872835322339,0.605457722909465));
#15505=CARTESIAN_POINT('Ctrl Pts',(9.1040197884667,-1.25519559703033,0.605388684776982));
#15506=CARTESIAN_POINT('Ctrl Pts',(8.20230020786566,-1.29401302889245,0.605326714446839));
#15507=CARTESIAN_POINT('Ctrl Pts',(7.29999999953094,-1.32031613471704,0.605285370449856));
#15508=CARTESIAN_POINT('Ctrl Pts',(10.4681436286308,-1.08420482079362,0.7));
#15509=CARTESIAN_POINT('Ctrl Pts',(10.3770124662346,-1.0891584122264,0.7));
#15510=CARTESIAN_POINT('Ctrl Pts',(10.285877616441,-1.09404209584202,0.7));
#15511=CARTESIAN_POINT('Ctrl Pts',(10.1947388861048,-1.09885088260188,0.7));
#15512=CARTESIAN_POINT('Ctrl Pts',(10.4697107510168,-1.11303515260326,0.7));
#15513=CARTESIAN_POINT('Ctrl Pts',(10.3785648662465,-1.11799094453753,0.700000051218742));
#15514=CARTESIAN_POINT('Ctrl Pts',(10.2874149314686,-1.12287675076168,0.699999949550842));
#15515=CARTESIAN_POINT('Ctrl Pts',(10.196260416419,-1.12768774893097,0.7));
#15516=CARTESIAN_POINT('Ctrl Pts',(10.4724269697127,-1.16300539549315,0.676698381019543));
#15517=CARTESIAN_POINT('Ctrl Pts',(10.3812557252598,-1.16796482352885,0.676696026813929));
#15518=CARTESIAN_POINT('Ctrl Pts',(10.2900793016129,-1.17285439035486,0.676693724638983));
#15519=CARTESIAN_POINT('Ctrl Pts',(10.1988975981852,-1.17766904563614,0.67669140632491));
#15520=CARTESIAN_POINT('Ctrl Pts',(10.4734985149421,-1.18271860027509,0.627116141711795));
#15521=CARTESIAN_POINT('Ctrl Pts',(10.382317043787,-1.18767684023183,0.627110048826767));
#15522=CARTESIAN_POINT('Ctrl Pts',(10.2911301919381,-1.19256517083271,0.627104033151799));
#15523=CARTESIAN_POINT('Ctrl Pts',(10.1999375452555,-1.19737868557977,0.627098033786781));
#15524=CARTESIAN_POINT('Ctrl Pts',(10.4735630903435,-1.18390659316268,0.605494180667944));
#15525=CARTESIAN_POINT('Ctrl Pts',(10.3823809652617,-1.18886335120032,0.605486986548286));
#15526=CARTESIAN_POINT('Ctrl Pts',(10.2911933328565,-1.19375025772558,0.605479840815741));
#15527=CARTESIAN_POINT('Ctrl Pts',(10.1999999975038,-1.19856231440453,0.605472757505366));
#15528=CARTESIAN_POINT('',(10.4681436258201,-1.08420482094639,0.7));
#15529=CARTESIAN_POINT('Ctrl Pts',(10.4681436258201,-1.0842048209464,0.7));
#15530=CARTESIAN_POINT('Ctrl Pts',(10.3787660248044,-1.08906309452597,0.7));
#15531=CARTESIAN_POINT('Ctrl Pts',(10.289384876933,-1.09385412476048,0.7));
#15532=CARTESIAN_POINT('Ctrl Pts',(10.1999999999973,-1.09857320510493,0.7));
#15533=CARTESIAN_POINT('Origin',(10.4681436286308,-1.08420482099672,0.6));
#15534=CARTESIAN_POINT('Origin',(5.4,-8.11656130105013E-18,0.7));
#15535=CARTESIAN_POINT('',(10.4681436286308,1.08420482109828,0.7));
#15536=CARTESIAN_POINT('Ctrl Pts',(10.1999999980461,1.09857320520795,0.7));
#15537=CARTESIAN_POINT('Ctrl Pts',(10.2893848765692,1.09385412478074,0.7));
#15538=CARTESIAN_POINT('Ctrl Pts',(10.3787660260279,1.08906309446088,0.7));
#15539=CARTESIAN_POINT('Ctrl Pts',(10.4681436286308,1.08420482079361,0.7));
#15540=CARTESIAN_POINT('',(10.4681436286308,0.7,0.7));
#15541=CARTESIAN_POINT('Ctrl Pts',(7.3,1.35236351479305,-3.57463069561303E-11));
#15542=CARTESIAN_POINT('Ctrl Pts',(7.29625341766908,1.34178092325856,0.20193409200674));
#15543=CARTESIAN_POINT('Ctrl Pts',(7.29250676907475,1.33119833465113,0.403868182976914));
#15544=CARTESIAN_POINT('Ctrl Pts',(7.28876005303626,1.32061574904014,0.60580227285657));
#15545=CARTESIAN_POINT('Ctrl Pts',(8.20875307682014,1.32613868191819,-8.19770140467192E-5));
#15546=CARTESIAN_POINT('Ctrl Pts',(8.20321812688841,1.31555630757352,0.201851960063995));
#15547=CARTESIAN_POINT('Ctrl Pts',(8.19768309032092,1.3049739355521,0.403785895138154));
#15548=CARTESIAN_POINT('Ctrl Pts',(8.19214796413082,1.29439157094932,0.605719828284144));
#15549=CARTESIAN_POINT('Ctrl Pts',(9.11786336174626,1.28732002675385,-0.000205293251048056));
#15550=CARTESIAN_POINT('Ctrl Pts',(9.11054075262572,1.27673792860073,0.201728409716354));
#15551=CARTESIAN_POINT('Ctrl Pts',(9.10321803982063,1.26615583517412,0.403662109357089));
#15552=CARTESIAN_POINT('Ctrl Pts',(9.09589522044026,1.25557375159787,0.605595805709147));
#15553=CARTESIAN_POINT('Ctrl Pts',(10.0273290644402,1.2407389515511,-0.000342977407187712));
#15554=CARTESIAN_POINT('Ctrl Pts',(10.0182194939295,1.23015709330624,0.201590462897949));
#15555=CARTESIAN_POINT('Ctrl Pts',(10.0091098064748,1.21957524432641,0.403523898424684));
#15556=CARTESIAN_POINT('Ctrl Pts',(10.,1.20899340483035,0.605457329091028));
#15557=CARTESIAN_POINT('Ctrl Pts',(10.2,1.23178301601276,-2.39624899783797E-11));
#15558=CARTESIAN_POINT('Ctrl Pts',(10.1905551755807,1.22120572247504,0.201847146346486));
#15559=CARTESIAN_POINT('Ctrl Pts',(10.1811102319479,1.21062843858352,0.403694287656288));
#15560=CARTESIAN_POINT('Ctrl Pts',(10.1716651669865,1.2000511645658,0.605541423818621));
#15561=CARTESIAN_POINT('Ctrl Pts',(10.3017512542641,1.22646400658951,-1.55944220863836E-5));
#15562=CARTESIAN_POINT('Ctrl Pts',(10.2921066085356,1.2158867394917,0.201831522196997));
#15563=CARTESIAN_POINT('Ctrl Pts',(10.2824618422272,1.20530948226672,0.403678633585648));
#15564=CARTESIAN_POINT('Ctrl Pts',(10.2728169531999,1.19473223514819,0.605525739654127));
#15565=CARTESIAN_POINT('Ctrl Pts',(10.4035069533242,1.22105168617711,-3.13468015701665E-5));
#15566=CARTESIAN_POINT('Ctrl Pts',(10.3936624949945,1.21047444506608,0.201815739750419));
#15567=CARTESIAN_POINT('Ctrl Pts',(10.3838179147698,1.19989721405077,0.40366282090032));
#15568=CARTESIAN_POINT('Ctrl Pts',(10.3739732104878,1.18931999337006,0.605509896555428));
#15569=CARTESIAN_POINT('Ctrl Pts',(10.5052670937653,1.21555282972323,-4.72191118859062E-5));
#15570=CARTESIAN_POINT('Ctrl Pts',(10.495222831523,1.20497561405169,0.201799837128814));
#15571=CARTESIAN_POINT('Ctrl Pts',(10.4851784461213,1.19439840869429,0.403646887794301));
#15572=CARTESIAN_POINT('Ctrl Pts',(10.4751339353761,1.18382121389426,0.605493932788864));
#15573=CARTESIAN_POINT('',(10.4735630903435,1.18390659316268,0.605494180667944));
#15574=CARTESIAN_POINT('Ctrl Pts',(10.5052647440597,1.21555035534119,-4.0462425077159E-16));
#15575=CARTESIAN_POINT('Ctrl Pts',(10.4946974680575,1.20500226999407,0.201831382381129));
#15576=CARTESIAN_POINT('Ctrl Pts',(10.4841302498201,1.19445434834508,0.40366277587515));
#15577=CARTESIAN_POINT('Ctrl Pts',(10.4735630903435,1.18390659316268,0.605494180667945));
#15578=CARTESIAN_POINT('Ctrl Pts',(10.4735630903435,1.18390659316268,0.605494180667944));
#15579=CARTESIAN_POINT('Ctrl Pts',(10.3823809652617,1.18886335120032,0.605486986548286));
#15580=CARTESIAN_POINT('Ctrl Pts',(10.2911933328565,1.19375025772558,0.605479840815741));
#15581=CARTESIAN_POINT('Ctrl Pts',(10.1999999975038,1.19856231440453,0.605472757505366));
#15582=CARTESIAN_POINT('Origin',(7.1,1.42555555555556,0.));
#15583=CARTESIAN_POINT('',(7.0999999994629,-1.32593912634735,0.605276549957215));
#15584=CARTESIAN_POINT('Ctrl Pts',(7.0999999994629,-1.32593912634735,0.605276549957215));
#15585=CARTESIAN_POINT('Ctrl Pts',(7.0999999994629,-1.33126650931098,0.504490734647167));
#15586=CARTESIAN_POINT('Ctrl Pts',(7.1,-1.33659376385849,0.403703958452373));
#15587=CARTESIAN_POINT('Ctrl Pts',(7.1,-1.3472576786761,0.201945747207886));
#15588=CARTESIAN_POINT('Ctrl Pts',(7.1,-1.35259443928223,0.100972400854069));
#15589=CARTESIAN_POINT('Ctrl Pts',(7.1,-1.35793097395724,0.));
#15590=CARTESIAN_POINT('',(7.1,-1.22604182196417,0.7));
#15591=CARTESIAN_POINT('Ctrl Pts',(7.1,-1.22604182196307,0.7));
#15592=CARTESIAN_POINT('Ctrl Pts',(7.1,-1.23395163718705,0.7));
#15593=CARTESIAN_POINT('Ctrl Pts',(7.09999945440688,-1.24179783218049,0.699006056038995));
#15594=CARTESIAN_POINT('Ctrl Pts',(7.09999897931553,-1.2494401870438,0.697119011207626));
#15595=CARTESIAN_POINT('Ctrl Pts',(7.09999871186578,-1.25374240366384,0.696056710937424));
#15596=CARTESIAN_POINT('Ctrl Pts',(7.09999846845149,-1.25798007942473,0.69471034534287));
#15597=CARTESIAN_POINT('Ctrl Pts',(7.09999831430822,-1.26212651101681,0.6930909329195));
#15598=CARTESIAN_POINT('Ctrl Pts',(7.09999803835695,-1.26954956016987,0.690191818885951));
#15599=CARTESIAN_POINT('Ctrl Pts',(7.09999810102228,-1.27659977900265,0.686452252582521));
#15600=CARTESIAN_POINT('Ctrl Pts',(7.09999845706054,-1.28313109767173,0.681953977461377));
#15601=CARTESIAN_POINT('Ctrl Pts',(7.09999865314126,-1.2867280867584,0.679476645189077));
#15602=CARTESIAN_POINT('Ctrl Pts',(7.09999893113315,-1.29016742765117,0.67676830886676));
#15603=CARTESIAN_POINT('Ctrl Pts',(7.09999917787259,-1.2934208019838,0.673837071833988));
#15604=CARTESIAN_POINT('Ctrl Pts',(7.09999941835505,-1.29659167515528,0.670980166997299));
#15605=CARTESIAN_POINT('Ctrl Pts',(7.09999963169439,-1.29956664557352,0.667928795646746));
#15606=CARTESIAN_POINT('Ctrl Pts',(7.09999963110542,-1.30232317314677,0.664694459428825));
#15607=CARTESIAN_POINT('Ctrl Pts',(7.09999963001387,-1.30743194453681,0.658700148145236));
#15608=CARTESIAN_POINT('Ctrl Pts',(7.09999897381858,-1.31179333085743,0.652078782729069));
#15609=CARTESIAN_POINT('Ctrl Pts',(7.09999874753952,-1.31534789998199,0.64499600756552));
#15610=CARTESIAN_POINT('Ctrl Pts',(7.09999872438549,-1.31571162172319,0.644271261689237));
#15611=CARTESIAN_POINT('Ctrl Pts',(7.0999987046402,-1.31606685549941,0.643541664816448));
#15612=CARTESIAN_POINT('Ctrl Pts',(7.09999868869212,-1.31641350913238,0.642807383257706));
#15613=CARTESIAN_POINT('Ctrl Pts',(7.09999853283271,-1.31980133087414,0.635631300872562));
#15614=CARTESIAN_POINT('Ctrl Pts',(7.09999885939544,-1.32233451509485,0.628092322434426));
#15615=CARTESIAN_POINT('Ctrl Pts',(7.09999934101855,-1.32395982399511,0.620358959365968));
#15616=CARTESIAN_POINT('Ctrl Pts',(7.09999964997549,-1.32500244522074,0.615398075635307));
#15617=CARTESIAN_POINT('Ctrl Pts',(7.09999999934316,-1.32567060646853,0.610356529630438));
#15618=CARTESIAN_POINT('Ctrl Pts',(7.09999999981141,-1.32593912630714,0.60527654995744));
#15619=CARTESIAN_POINT('',(7.09999999995537,1.22604182196549,0.7));
#15620=CARTESIAN_POINT('',(7.1,0.712777777777778,0.7));
#15621=CARTESIAN_POINT('',(7.0999999994629,1.32593912634735,0.605276549957215));
#15622=CARTESIAN_POINT('Ctrl Pts',(7.09999999981142,1.32593912630714,0.60527654995744));
#15623=CARTESIAN_POINT('Ctrl Pts',(7.09999999908198,1.32552083177145,0.613190035045322));
#15624=CARTESIAN_POINT('Ctrl Pts',(7.09999922367565,1.32413525001942,0.621012727860624));
#15625=CARTESIAN_POINT('Ctrl Pts',(7.09999888117586,1.32186630199077,0.628584136488803));
#15626=CARTESIAN_POINT('Ctrl Pts',(7.09999868987568,1.32059900146923,0.632813078704371));
#15627=CARTESIAN_POINT('Ctrl Pts',(7.09999860640034,1.3190551184949,0.636963663611311));
#15628=CARTESIAN_POINT('Ctrl Pts',(7.09999865766138,1.31724253497577,0.641005923298765));
#15629=CARTESIAN_POINT('Ctrl Pts',(7.0999987494091,1.31399834762864,0.648240816253195));
#15630=CARTESIAN_POINT('Ctrl Pts',(7.09999933613984,1.30993159792479,0.655050690394837));
#15631=CARTESIAN_POINT('Ctrl Pts',(7.09999956222935,1.30510592187917,0.661272231165006));
#15632=CARTESIAN_POINT('Ctrl Pts',(7.09999960444598,1.30420484616769,0.662433950108221));
#15633=CARTESIAN_POINT('Ctrl Pts',(7.09999963060969,1.30327718139331,0.663575086117144));
#15634=CARTESIAN_POINT('Ctrl Pts',(7.09999963056866,1.30232317316131,0.664694459428815));
#15635=CARTESIAN_POINT('Ctrl Pts',(7.09999963048683,1.30042028596585,0.666927187690779));
#15636=CARTESIAN_POINT('Ctrl Pts',(7.09999952705857,1.29841262431024,0.669073382394206));
#15637=CARTESIAN_POINT('Ctrl Pts',(7.09999938633452,1.29630755303174,0.671129253595323));
#15638=CARTESIAN_POINT('Ctrl Pts',(7.09999900634735,1.29062337821964,0.676680576924663));
#15639=CARTESIAN_POINT('Ctrl Pts',(7.09999841760642,1.2842958957007,0.681513596217188));
#15640=CARTESIAN_POINT('Ctrl Pts',(7.0999982224057,1.2774887935492,0.68557385059291));
#15641=CARTESIAN_POINT('Ctrl Pts',(7.09999809840912,1.27316474526651,0.688153029745784));
#15642=CARTESIAN_POINT('Ctrl Pts',(7.09999810738417,1.26864620899217,0.690419707112974));
#15643=CARTESIAN_POINT('Ctrl Pts',(7.09999825155258,1.26396949224645,0.69235064530212));
#15644=CARTESIAN_POINT('Ctrl Pts',(7.09999847710269,1.25665281355793,0.695371579659609));
#15645=CARTESIAN_POINT('Ctrl Pts',(7.09999903441007,1.2490339950321,0.697538299034574));
#15646=CARTESIAN_POINT('Ctrl Pts',(7.09999948258254,1.24125996729125,0.698781081437474));
#15647=CARTESIAN_POINT('Ctrl Pts',(7.09999977198436,1.23623998534067,0.699583592753232));
#15648=CARTESIAN_POINT('Ctrl Pts',(7.1,1.23115469319345,0.7));
#15649=CARTESIAN_POINT('Ctrl Pts',(7.1,1.22604182196307,0.7));
#15650=CARTESIAN_POINT('Ctrl Pts',(7.1,1.35793097395724,0.));
#15651=CARTESIAN_POINT('Ctrl Pts',(7.1,1.35259441576718,0.100972845781549));
#15652=CARTESIAN_POINT('Ctrl Pts',(7.1,1.34725763161617,0.201946637598055));
#15653=CARTESIAN_POINT('Ctrl Pts',(7.1,1.33659371676552,0.403704849408333));
#15654=CARTESIAN_POINT('Ctrl Pts',(7.0999999994629,1.33126648576411,0.504491180117376));
#15655=CARTESIAN_POINT('Ctrl Pts',(7.0999999994629,1.32593912634735,0.605276549957215));
#15656=CARTESIAN_POINT('Ctrl Pts',(7.11011156210589,-1.35766432821499,-9.27062925672982E-5));
#15657=CARTESIAN_POINT('Ctrl Pts',(7.10674110347764,-1.34708925835705,0.201697046690488));
#15658=CARTESIAN_POINT('Ctrl Pts',(7.10337058314201,-1.33651419103807,0.403486798779133));
#15659=CARTESIAN_POINT('Ctrl Pts',(7.09999999999996,-1.32593912631822,0.605276549958221));
#15660=CARTESIAN_POINT('Ctrl Pts',(5.9694837631095,-1.38835096090528,2.80675674898241E-6));
#15661=CARTESIAN_POINT('Ctrl Pts',(5.96835662351021,-1.37777563343505,0.201792740207853));
#15662=CARTESIAN_POINT('Ctrl Pts',(5.96722945517891,-1.3672003004237,0.40358267322573));
#15663=CARTESIAN_POINT('Ctrl Pts',(5.96610224583462,-1.35662497356325,0.605372606931572));
#15664=CARTESIAN_POINT('Ctrl Pts',(4.8294200007394,-1.39866452387306,3.01102374082134E-5));
#15665=CARTESIAN_POINT('Ctrl Pts',(4.83053730380309,-1.38808904115766,0.201820093264151));
#15666=CARTESIAN_POINT('Ctrl Pts',(4.83165461298617,-1.3775135517806,0.403610075973038));
#15667=CARTESIAN_POINT('Ctrl Pts',(4.83277191472125,-1.36693806692183,0.605400059795761));
#15668=CARTESIAN_POINT('Ctrl Pts',(3.68991216363982,-1.37907703205181,-6.2684699445455E-5));
#15669=CARTESIAN_POINT('Ctrl Pts',(3.69327498756969,-1.36850179198701,0.201727122618256));
#15670=CARTESIAN_POINT('Ctrl Pts',(3.69663785098144,-1.3579265529724,0.403516929334346));
#15671=CARTESIAN_POINT('Ctrl Pts',(3.70000075457889,-1.34735131503281,0.605306735438421));
#15672=CARTESIAN_POINT('Ctrl Pts',(3.69999999992215,-1.34735368792773,0.6052614572053));
#15673=CARTESIAN_POINT('Ctrl Pts',(4.83355316856959,-1.366961322855,0.605214762857233));
#15674=CARTESIAN_POINT('Ctrl Pts',(5.96724522208681,-1.35660163688233,0.605228569880684));
#15675=CARTESIAN_POINT('Ctrl Pts',(7.09999999927392,-1.32593912632169,0.605276549957417));
#15676=CARTESIAN_POINT('Ctrl Pts',(7.1,-1.22604182196307,0.7));
#15677=CARTESIAN_POINT('Ctrl Pts',(5.96696284938742,-1.25674179781664,0.7));
#15678=CARTESIAN_POINT('Ctrl Pts',(4.83327074934872,-1.26710800714677,0.7));
#15679=CARTESIAN_POINT('Ctrl Pts',(3.7,-1.24747724070879,0.7));
#15680=CARTESIAN_POINT('Ctrl Pts',(7.10078315634008,-1.25494559805327,0.7));
#15681=CARTESIAN_POINT('Ctrl Pts',(5.96739926106349,-1.28566432005869,0.700000343763215));
#15682=CARTESIAN_POINT('Ctrl Pts',(4.83328164159484,-1.29603890521481,0.700000334703603));
#15683=CARTESIAN_POINT('Ctrl Pts',(3.69949916377151,-1.27639017438114,0.7));
#15684=CARTESIAN_POINT('Ctrl Pts',(7.10214055788579,-1.30504291366416,0.676629771601708));
#15685=CARTESIAN_POINT('Ctrl Pts',(5.96815960929481,-1.33579288254824,0.676614006760374));
#15686=CARTESIAN_POINT('Ctrl Pts',(4.83329467960724,-1.3461818279488,0.676609489640654));
#15687=CARTESIAN_POINT('Ctrl Pts',(3.69863109538965,-1.3265031696486,0.676624836591801));
#15688=CARTESIAN_POINT('Ctrl Pts',(7.10267376869946,-1.32472200604796,0.626932241521275));
#15689=CARTESIAN_POINT('Ctrl Pts',(5.9684558952243,-1.35546668061705,0.626891484245174));
#15690=CARTESIAN_POINT('Ctrl Pts',(4.83330292199863,-1.36585610284781,0.626879766983475));
#15691=CARTESIAN_POINT('Ctrl Pts',(3.69829020046733,-1.34618280086838,0.626919440930842));
#15692=CARTESIAN_POINT('Ctrl Pts',(7.10270476209941,-1.32586587253612,0.605276664588022));
#15693=CARTESIAN_POINT('Ctrl Pts',(5.96847377630401,-1.35660073810322,0.605228567467576));
#15694=CARTESIAN_POINT('Ctrl Pts',(4.8333022084086,-1.36698748587873,0.605214711607465));
#15695=CARTESIAN_POINT('Ctrl Pts',(3.69827043673666,-1.34732374755196,0.60526152849799));
#15696=CARTESIAN_POINT('Ctrl Pts',(7.1,-1.22604182196307,0.7));
#15697=CARTESIAN_POINT('Ctrl Pts',(5.96696284938742,-1.25674179781664,0.7));
#15698=CARTESIAN_POINT('Ctrl Pts',(4.83327074934872,-1.26710800714677,0.7));
#15699=CARTESIAN_POINT('Ctrl Pts',(3.7,-1.24747724070879,0.7));
#15700=CARTESIAN_POINT('Origin',(5.4,-8.11656130105013E-18,0.7));
#15701=CARTESIAN_POINT('Ctrl Pts',(3.7,1.24747724070879,0.7));
#15702=CARTESIAN_POINT('Ctrl Pts',(4.83327074934871,1.26710800714677,0.7));
#15703=CARTESIAN_POINT('Ctrl Pts',(5.96696284938742,1.25674179781664,0.7));
#15704=CARTESIAN_POINT('Ctrl Pts',(7.1,1.22604182196307,0.7));
#15705=CARTESIAN_POINT('Ctrl Pts',(3.7,1.24747724070879,0.7));
#15706=CARTESIAN_POINT('Ctrl Pts',(4.83327074934871,1.26710800714677,0.7));
#15707=CARTESIAN_POINT('Ctrl Pts',(5.96696284938742,1.25674179781664,0.7));
#15708=CARTESIAN_POINT('Ctrl Pts',(7.1,1.22604182196307,0.7));
#15709=CARTESIAN_POINT('Ctrl Pts',(3.69949916377151,1.27639017438114,0.7));
#15710=CARTESIAN_POINT('Ctrl Pts',(4.83328164159484,1.29603890521481,0.700000334703603));
#15711=CARTESIAN_POINT('Ctrl Pts',(5.96739926106349,1.28566432005869,0.700000343763215));
#15712=CARTESIAN_POINT('Ctrl Pts',(7.10078315634008,1.25494559805327,0.7));
#15713=CARTESIAN_POINT('Ctrl Pts',(3.69863109538965,1.3265031696486,0.676624836591801));
#15714=CARTESIAN_POINT('Ctrl Pts',(4.83329467960724,1.3461818279488,0.676609489640654));
#15715=CARTESIAN_POINT('Ctrl Pts',(5.9681596092948,1.33579288254824,0.676614006760374));
#15716=CARTESIAN_POINT('Ctrl Pts',(7.10214055788579,1.30504291366416,0.676629771601707));
#15717=CARTESIAN_POINT('Ctrl Pts',(3.69829020046733,1.34618280086838,0.626919440930842));
#15718=CARTESIAN_POINT('Ctrl Pts',(4.83330292199863,1.36585610284781,0.626879766983475));
#15719=CARTESIAN_POINT('Ctrl Pts',(5.9684558952243,1.35546668061705,0.626891484245174));
#15720=CARTESIAN_POINT('Ctrl Pts',(7.10267376869946,1.32472200604796,0.626932241521275));
#15721=CARTESIAN_POINT('Ctrl Pts',(3.69827043673666,1.34732374755196,0.60526152849799));
#15722=CARTESIAN_POINT('Ctrl Pts',(4.83330220840859,1.36698748587873,0.605214711607465));
#15723=CARTESIAN_POINT('Ctrl Pts',(5.96847377630401,1.35660073810322,0.605228567467576));
#15724=CARTESIAN_POINT('Ctrl Pts',(7.10270476209941,1.32586587253612,0.605276664588022));
#15725=CARTESIAN_POINT('Ctrl Pts',(7.09999999927392,1.32593912632169,0.605276549957417));
#15726=CARTESIAN_POINT('Ctrl Pts',(5.96724522208681,1.35660163688233,0.605228569880684));
#15727=CARTESIAN_POINT('Ctrl Pts',(4.83355316856959,1.366961322855,0.605214762857233));
#15728=CARTESIAN_POINT('Ctrl Pts',(3.69999999992215,1.34735368792773,0.6052614572053));
#15729=CARTESIAN_POINT('Ctrl Pts',(3.68991216360307,1.37907703216746,-6.26869063400631E-5));
#15730=CARTESIAN_POINT('Ctrl Pts',(3.6932749875452,1.36850179206412,0.201727121146993));
#15731=CARTESIAN_POINT('Ctrl Pts',(3.69663785096921,1.35792655301095,0.403516928598715));
#15732=CARTESIAN_POINT('Ctrl Pts',(3.70000075457892,1.34735131503281,0.605306735438421));
#15733=CARTESIAN_POINT('Ctrl Pts',(4.8294200007272,1.39866452398872,3.01080305115927E-5));
#15734=CARTESIAN_POINT('Ctrl Pts',(4.83053730379496,1.38808904123477,0.201820091792887));
#15735=CARTESIAN_POINT('Ctrl Pts',(4.83165461298211,1.37751355181915,0.403610075237406));
#15736=CARTESIAN_POINT('Ctrl Pts',(4.83277191472127,1.36693806692183,0.605400059795761));
#15737=CARTESIAN_POINT('Ctrl Pts',(5.96948376312183,1.38835096102094,2.80454985295556E-6));
#15738=CARTESIAN_POINT('Ctrl Pts',(5.96835662351844,1.37777563351215,0.201792738736588));
#15739=CARTESIAN_POINT('Ctrl Pts',(5.96722945518303,1.36720030046225,0.403582672490098));
#15740=CARTESIAN_POINT('Ctrl Pts',(5.96610224583462,1.35662497356325,0.605372606931572));
#15741=CARTESIAN_POINT('Ctrl Pts',(7.11011156214274,1.35766432833065,-9.27084994613511E-5));
#15742=CARTESIAN_POINT('Ctrl Pts',(7.10674110350221,1.34708925843416,0.201697045219225));
#15743=CARTESIAN_POINT('Ctrl Pts',(7.10337058315429,1.33651419107662,0.403486798043502));
#15744=CARTESIAN_POINT('Ctrl Pts',(7.09999999999996,1.32593912631822,0.605276549958221));
#15745=CARTESIAN_POINT('Origin',(3.5,1.44777777777778,0.));
#15746=CARTESIAN_POINT('',(3.5,-1.34358136363184,0.605270327458634));
#15747=CARTESIAN_POINT('Ctrl Pts',(3.5,-1.34358136363184,0.605270327458634));
#15748=CARTESIAN_POINT('Ctrl Pts',(3.5,-1.34890136370362,0.504489156176152));
#15749=CARTESIAN_POINT('Ctrl Pts',(3.5,-1.35422123464986,0.403706701640381));
#15750=CARTESIAN_POINT('Ctrl Pts',(3.5,-1.3648706701715,0.201950780690867));
#15751=CARTESIAN_POINT('Ctrl Pts',(3.5,-1.3702003690246,0.100974756199658));
#15752=CARTESIAN_POINT('Ctrl Pts',(3.5,-1.37552980833516,0.));
#15753=CARTESIAN_POINT('',(3.5,-1.24369946473884,0.7));
#15754=CARTESIAN_POINT('Ctrl Pts',(3.49999999991873,-1.24369946470729,0.7));
#15755=CARTESIAN_POINT('Ctrl Pts',(3.49999999896975,-1.25160831520001,0.699999999810925));
#15756=CARTESIAN_POINT('Ctrl Pts',(3.50000040534574,-1.25945374057332,0.69900619751828));
#15757=CARTESIAN_POINT('Ctrl Pts',(3.50000075715473,-1.26709539726361,0.697119355224275));
#15758=CARTESIAN_POINT('Ctrl Pts',(3.5000009551612,-1.27139630362835,0.696057395447694));
#15759=CARTESIAN_POINT('Ctrl Pts',(3.50000113454144,-1.27563271975905,0.694711510656402));
#15760=CARTESIAN_POINT('Ctrl Pts',(3.50000124621709,-1.27977793997275,0.693092697679401));
#15761=CARTESIAN_POINT('Ctrl Pts',(3.50000144618968,-1.28720060051191,0.690193961644836));
#15762=CARTESIAN_POINT('Ctrl Pts',(3.50000138985083,-1.29425038514255,0.686454755369034));
#15763=CARTESIAN_POINT('Ctrl Pts',(3.5000011147959,-1.30078112659466,0.681956784255818));
#15764=CARTESIAN_POINT('Ctrl Pts',(3.50000096334461,-1.30437709646577,0.679480102439082));
#15765=CARTESIAN_POINT('Ctrl Pts',(3.50000075087427,-1.30781543681835,0.676772489296601));
#15766=CARTESIAN_POINT('Ctrl Pts',(3.50000056308077,-1.31106783354026,0.67384203444854));
#15767=CARTESIAN_POINT('Ctrl Pts',(3.50000037990614,-1.31424023611357,0.670983655445047));
#15768=CARTESIAN_POINT('Ctrl Pts',(3.50000021841608,-1.31721646102264,0.667930553458483));
#15769=CARTESIAN_POINT('Ctrl Pts',(3.50000022028926,-1.3199739184757,0.664694242102541));
#15770=CARTESIAN_POINT('Ctrl Pts',(3.50000022375892,-1.32508151834405,0.658699667848218));
#15771=CARTESIAN_POINT('Ctrl Pts',(3.50000072745304,-1.32944146850927,0.652077914129702));
#15772=CARTESIAN_POINT('Ctrl Pts',(3.50000090782832,-1.33299465793893,0.64499486611401));
#15773=CARTESIAN_POINT('Ctrl Pts',(3.50000092626355,-1.33335781125732,0.644270944003422));
#15774=CARTESIAN_POINT('Ctrl Pts',(3.50000094214549,-1.33371249714824,0.643542183465449));
#15775=CARTESIAN_POINT('Ctrl Pts',(3.5000009551778,-1.33405862411533,0.642808750463418));
#15776=CARTESIAN_POINT('Ctrl Pts',(3.50000108270827,-1.3374457225345,0.635631587173848));
#15777=CARTESIAN_POINT('Ctrl Pts',(3.5000008470667,-1.33997810357527,0.628091493562486));
#15778=CARTESIAN_POINT('Ctrl Pts',(3.50000049017339,-1.34160279315579,0.620357239364781));
#15779=CARTESIAN_POINT('Ctrl Pts',(3.50000026118253,-1.3426452308862,0.615394766232079));
#15780=CARTESIAN_POINT('Ctrl Pts',(3.5,-1.34331313055125,0.610351689051435));
#15781=CARTESIAN_POINT('Ctrl Pts',(3.5,-1.34358136363184,0.605270327458634));
#15782=CARTESIAN_POINT('',(3.5,0.723888888888889,0.7));
#15783=CARTESIAN_POINT('Ctrl Pts',(3.5,1.37552980833516,0.));
#15784=CARTESIAN_POINT('Ctrl Pts',(3.5,1.37020035376703,0.10097504527886));
#15785=CARTESIAN_POINT('Ctrl Pts',(3.5,1.36487063968137,0.201951358354439));
#15786=CARTESIAN_POINT('Ctrl Pts',(3.5,1.35422120417274,0.403707279015233));
#15787=CARTESIAN_POINT('Ctrl Pts',(3.5,1.34890134846466,0.504489444860456));
#15788=CARTESIAN_POINT('Ctrl Pts',(3.5,1.34358136363184,0.605270327458635));
#15789=CARTESIAN_POINT('Ctrl Pts',(3.50000000097418,-1.37552980835478,3.46944695195361E-18));
#15790=CARTESIAN_POINT('Ctrl Pts',(3.50374047168104,-1.36494504174376,0.201972406882836));
#15791=CARTESIAN_POINT('Ctrl Pts',(3.50748098869546,-1.35436027657305,0.403944812985359));
#15792=CARTESIAN_POINT('Ctrl Pts',(3.51122155284351,-1.34377551287676,0.605917218294091));
#15793=CARTESIAN_POINT('Ctrl Pts',(2.69119625874569,-1.35924722858667,-7.54309614812119E-5));
#15794=CARTESIAN_POINT('Ctrl Pts',(2.69653217397324,-1.34866266892899,0.20189683354744));
#15795=CARTESIAN_POINT('Ctrl Pts',(2.70186816749714,-1.3380781117335,0.403869096002786));
#15796=CARTESIAN_POINT('Ctrl Pts',(2.7072042346663,-1.32749355863083,0.605841357314298));
#15797=CARTESIAN_POINT('Ctrl Pts',(1.88267190563219,-1.32763345268679,-0.000212792412547521));
#15798=CARTESIAN_POINT('Ctrl Pts',(1.88960380459144,-1.31704931403188,0.201759213581099));
#15799=CARTESIAN_POINT('Ctrl Pts',(1.89653581411498,-1.30646518166523,0.403731216009517));
#15800=CARTESIAN_POINT('Ctrl Pts',(1.90346792975642,-1.29588105699583,0.605703215867581));
#15801=CARTESIAN_POINT('Ctrl Pts',(1.07441451989529,-1.27728918272486,-0.000429194541766893));
#15802=CARTESIAN_POINT('Ctrl Pts',(1.08294287068452,-1.26670581246828,0.201542410257184));
#15803=CARTESIAN_POINT('Ctrl Pts',(1.09147136321593,-1.25612245578053,0.403514009799157));
#15804=CARTESIAN_POINT('Ctrl Pts',(1.09999999999989,-1.24553911298205,0.605485603995245));
#15805=CARTESIAN_POINT('Ctrl Pts',(1.09999999916631,-1.24553911263844,0.605485603997431));
#15806=CARTESIAN_POINT('Ctrl Pts',(1.89930203168262,-1.29563783986497,0.605377360150118));
#15807=CARTESIAN_POINT('Ctrl Pts',(2.69958486793449,-1.32722445934619,0.605308375488923));
#15808=CARTESIAN_POINT('Ctrl Pts',(3.5,-1.34358136363184,0.605270327458634));
#15809=CARTESIAN_POINT('Ctrl Pts',(3.50204003610941,-1.24374118183538,0.7));
#15810=CARTESIAN_POINT('Ctrl Pts',(2.70080437300401,-1.2273695200909,0.7));
#15811=CARTESIAN_POINT('Ctrl Pts',(1.89984199608574,-1.1957170361627,0.7));
#15812=CARTESIAN_POINT('Ctrl Pts',(1.1,-1.14549341399196,0.7));
#15813=CARTESIAN_POINT('Ctrl Pts',(3.50144932661635,-1.27265074030048,0.7));
#15814=CARTESIAN_POINT('Ctrl Pts',(2.6998452019678,-1.25626413437997,0.699999727319846));
#15815=CARTESIAN_POINT('Ctrl Pts',(1.89847848223078,-1.22458382597074,0.70000077422621));
#15816=CARTESIAN_POINT('Ctrl Pts',(1.09819048660397,-1.17431102498992,0.7));
#15817=CARTESIAN_POINT('Ctrl Pts',(3.50042536655637,-1.322763754511,0.676632802377821));
#15818=CARTESIAN_POINT('Ctrl Pts',(2.69818680938114,-1.3063522351595,0.67664530655333));
#15819=CARTESIAN_POINT('Ctrl Pts',(1.89610976425884,-1.27462253270773,0.67666760713801));
#15820=CARTESIAN_POINT('Ctrl Pts',(1.09505363188407,-1.22426736091617,0.676703190608825));
#15821=CARTESIAN_POINT('Ctrl Pts',(3.50002334924346,-1.34243864233338,0.626926882269943));
#15822=CARTESIAN_POINT('Ctrl Pts',(2.6975332861013,-1.32603127467068,0.626959208652505));
#15823=CARTESIAN_POINT('Ctrl Pts',(1.89518106151152,-1.29430885982199,0.62701751976321));
#15824=CARTESIAN_POINT('Ctrl Pts',(1.09381704710221,-1.24396073223232,0.627109609335854));
#15825=CARTESIAN_POINT('Ctrl Pts',(3.5,-1.34358136363184,0.605270327458634));
#15826=CARTESIAN_POINT('Ctrl Pts',(2.69749615303,-1.32718177535833,0.605308474776761));
#15827=CARTESIAN_POINT('Ctrl Pts',(1.89512529323683,-1.29547288309274,0.605377720397184));
#15828=CARTESIAN_POINT('Ctrl Pts',(1.09374258853658,-1.24514653057163,0.605486452199395));
#15829=CARTESIAN_POINT('Ctrl Pts',(3.49999999991875,-1.24369946470729,0.7));
#15830=CARTESIAN_POINT('Ctrl Pts',(3.26917843083003,-1.23897560807887,0.7));
#15831=CARTESIAN_POINT('Ctrl Pts',(3.03837960179139,-1.23298334389983,0.7));
#15832=CARTESIAN_POINT('Ctrl Pts',(2.80762376541487,-1.22564400623233,0.7));
#15833=CARTESIAN_POINT('Ctrl Pts',(2.57739190516312,-1.2178709162388,0.7));
#15834=CARTESIAN_POINT('Ctrl Pts',(2.08463535466707,-1.20026407570248,0.7));
#15835=CARTESIAN_POINT('Ctrl Pts',(1.59210562457525,-1.17639367564078,0.7));
#15836=CARTESIAN_POINT('Ctrl Pts',(1.1,-1.14549341399196,0.7));
#15837=CARTESIAN_POINT('Origin',(5.4,-8.11656130105013E-18,0.7));
#15838=CARTESIAN_POINT('Ctrl Pts',(1.0744145198953,1.27728918272486,-0.000429194541767127));
#15839=CARTESIAN_POINT('Ctrl Pts',(1.08294287068452,1.26670581246828,0.201542410257184));
#15840=CARTESIAN_POINT('Ctrl Pts',(1.09147136321593,1.25612245578053,0.403514009799157));
#15841=CARTESIAN_POINT('Ctrl Pts',(1.0999999999999,1.24553911298205,0.605485603995245));
#15842=CARTESIAN_POINT('Ctrl Pts',(1.88267190563235,1.3276334526868,-0.000212792412547728));
#15843=CARTESIAN_POINT('Ctrl Pts',(1.8896038045916,1.31704931403189,0.201759213581098));
#15844=CARTESIAN_POINT('Ctrl Pts',(1.89653581411514,1.30646518166524,0.403731216009517));
#15845=CARTESIAN_POINT('Ctrl Pts',(1.90346792975658,1.29588105699584,0.605703215867581));
#15846=CARTESIAN_POINT('Ctrl Pts',(2.69119625874601,1.35924722858668,-7.54309614812134E-5));
#15847=CARTESIAN_POINT('Ctrl Pts',(2.69653217397356,1.348662668929,0.201896833547441));
#15848=CARTESIAN_POINT('Ctrl Pts',(2.70186816749745,1.33807811173351,0.403869096002786));
#15849=CARTESIAN_POINT('Ctrl Pts',(2.70720423466661,1.32749355863085,0.605841357314298));
#15850=CARTESIAN_POINT('Ctrl Pts',(3.50000000097466,1.37552980835479,-3.81639164714898E-17));
#15851=CARTESIAN_POINT('Ctrl Pts',(3.50374047168151,1.36494504174377,0.201972406882836));
#15852=CARTESIAN_POINT('Ctrl Pts',(3.50748098869594,1.35436027657306,0.403944812985359));
#15853=CARTESIAN_POINT('Ctrl Pts',(3.51122155284398,1.34377551287677,0.605917218294091));
#15854=CARTESIAN_POINT('Origin',(0.9,1.34328341716202,0.));
#15855=CARTESIAN_POINT('',(0.9,-1.23261418131727,0.605513513251856));
#15856=CARTESIAN_POINT('Ctrl Pts',(0.9,-1.23261418131727,0.605513513251856));
#15857=CARTESIAN_POINT('Ctrl Pts',(0.9,-1.23820195798151,0.504544236118289));
#15858=CARTESIAN_POINT('Ctrl Pts',(0.9,-1.24378834611607,0.403573587101897));
#15859=CARTESIAN_POINT('Ctrl Pts',(0.9,-1.25495246062481,0.201736610752668));
#15860=CARTESIAN_POINT('Ctrl Pts',(0.9,-1.26053033259331,0.100867703930409));
#15861=CARTESIAN_POINT('Ctrl Pts',(0.9,-1.266106713614,0.));
#15862=CARTESIAN_POINT('',(0.9,-1.13254484134404,0.7));
#15863=CARTESIAN_POINT('Ctrl Pts',(0.899999999937205,-1.13254484130906,
0.7));
#15864=CARTESIAN_POINT('Ctrl Pts',(0.899999996287105,-1.14047016437301,
0.699999998205918));
#15865=CARTESIAN_POINT('Ctrl Pts',(0.900001280561548,-1.14833327216777,
0.699006663725481));
#15866=CARTESIAN_POINT('Ctrl Pts',(0.900002371513522,-1.15599299513142,
0.697119896446058));
#15867=CARTESIAN_POINT('Ctrl Pts',(0.900002982478546,-1.16028266409831,
0.696063251566776));
#15868=CARTESIAN_POINT('Ctrl Pts',(0.900003528700818,-1.16450859688491,
0.694725368779139));
#15869=CARTESIAN_POINT('Ctrl Pts',(0.900003857331964,-1.16864431737637,
0.693116947675672));
#15870=CARTESIAN_POINT('Ctrl Pts',(0.900004447924614,-1.17607674172948,
0.690226407030055));
#15871=CARTESIAN_POINT('Ctrl Pts',(0.900004211500339,-1.18313828052408,
0.686496282267003));
#15872=CARTESIAN_POINT('Ctrl Pts',(0.900003280035406,-1.18968205680082,
0.682006679400108));
#15873=CARTESIAN_POINT('Ctrl Pts',(0.900002768383153,-1.19327654302499,
0.679540547464272));
#15874=CARTESIAN_POINT('Ctrl Pts',(0.900002064672634,-1.19671453445753,
0.676844382327844));
#15875=CARTESIAN_POINT('Ctrl Pts',(0.900001450170085,-1.19996775918788,
0.673925988054463));
#15876=CARTESIAN_POINT('Ctrl Pts',(0.900000850201302,-1.20314404102283,
0.67107661751105));
#15877=CARTESIAN_POINT('Ctrl Pts',(0.900000329673364,-1.20612495630093,
0.668032594545539));
#15878=CARTESIAN_POINT('Ctrl Pts',(0.900000346081477,-1.20888784276431,
0.664805176146368));
#15879=CARTESIAN_POINT('Ctrl Pts',(0.900000376514472,-1.21401231436848,
0.658819112599938));
#15880=CARTESIAN_POINT('Ctrl Pts',(0.900002057232535,-1.21838968018573,
0.652203523053766));
#15881=CARTESIAN_POINT('Ctrl Pts',(0.900002698394847,-1.22195969054856,
0.645123732731769));
#15882=CARTESIAN_POINT('Ctrl Pts',(0.900002763240662,-1.22232075393107,
0.644407697543824));
#15883=CARTESIAN_POINT('Ctrl Pts',(0.90000282009371,-1.22267351953901,0.643686895083047));
#15884=CARTESIAN_POINT('Ctrl Pts',(0.900002868017411,-1.22301789747605,
0.642961485862499));
#15885=CARTESIAN_POINT('Ctrl Pts',(0.900003341628975,-1.22642125256928,
0.635792544708285));
#15886=CARTESIAN_POINT('Ctrl Pts',(0.900002645022176,-1.22896979279554,
0.628258742918086));
#15887=CARTESIAN_POINT('Ctrl Pts',(0.900001532827652,-1.23061007098772,
0.6205286650049));
#15888=CARTESIAN_POINT('Ctrl Pts',(0.900000822323555,-1.23165793118585,
0.61559045329652));
#15889=CARTESIAN_POINT('Ctrl Pts',(0.900000000000001,-1.23233426661673,
0.610571479357261));
#15890=CARTESIAN_POINT('Ctrl Pts',(0.900000000000001,-1.23261418131727,
0.605513513251856));
#15891=CARTESIAN_POINT('',(0.9,1.13254484134404,0.7));
#15892=CARTESIAN_POINT('',(0.9,0.671641708581009,0.7));
#15893=CARTESIAN_POINT('',(0.9,1.23261418131727,0.605513513251856));
#15894=CARTESIAN_POINT('Ctrl Pts',(0.9,1.23261418131727,0.605513513251856));
#15895=CARTESIAN_POINT('Ctrl Pts',(0.9,1.23217633603244,0.613425232807268));
#15896=CARTESIAN_POINT('Ctrl Pts',(0.900001832787994,1.23077105609892,0.621244170085157));
#15897=CARTESIAN_POINT('Ctrl Pts',(0.900002580745575,1.22848219166492,0.628809599741497));
#15898=CARTESIAN_POINT('Ctrl Pts',(0.900002993068559,1.22722042035689,0.632980157827643));
#15899=CARTESIAN_POINT('Ctrl Pts',(0.90000314174678,1.22568915198244,0.637073706995481));
#15900=CARTESIAN_POINT('Ctrl Pts',(0.900002971484041,1.2238959908032,0.641061424759933));
#15901=CARTESIAN_POINT('Ctrl Pts',(0.900002662567364,1.22064256379503,0.648296551655426));
#15902=CARTESIAN_POINT('Ctrl Pts',(0.900001146653719,1.21656554418039,0.655104870690721));
#15903=CARTESIAN_POINT('Ctrl Pts',(0.900000540233788,1.21172928299109,0.66132323772617));
#15904=CARTESIAN_POINT('Ctrl Pts',(0.900000424918953,1.21080963534652,0.66250570210793));
#15905=CARTESIAN_POINT('Ctrl Pts',(0.900000351402035,1.20986240082127,0.663666762843393));
#15906=CARTESIAN_POINT('Ctrl Pts',(0.900000346234225,1.20888784277449,0.664805176146358));
#15907=CARTESIAN_POINT('Ctrl Pts',(0.900000336405833,1.20703438079614,0.666970266034709));
#15908=CARTESIAN_POINT('Ctrl Pts',(0.900000571869483,1.20508211779724,0.669053482241208));
#15909=CARTESIAN_POINT('Ctrl Pts',(0.900000903580486,1.20303784749416,0.671051418948595));
#15910=CARTESIAN_POINT('Ctrl Pts',(0.900001825932764,1.19735357006848,0.676606861644505));
#15911=CARTESIAN_POINT('Ctrl Pts',(0.900003332967427,1.19102482074992,0.681443262092019));
#15912=CARTESIAN_POINT('Ctrl Pts',(0.900003895332687,1.18421635668109,0.685507797106414));
#15913=CARTESIAN_POINT('Ctrl Pts',(0.900004254598985,1.17986677848026,0.688104419886002));
#15914=CARTESIAN_POINT('Ctrl Pts',(0.9000042929279,1.17532044218795,0.69038534615497));
#15915=CARTESIAN_POINT('Ctrl Pts',(0.900003997675654,1.17061445353731,0.692327416690341));
#15916=CARTESIAN_POINT('Ctrl Pts',(0.900003537640084,1.16328200409216,0.695353376818313));
#15917=CARTESIAN_POINT('Ctrl Pts',(0.900002259964378,1.15564663185935,0.697524398440697));
#15918=CARTESIAN_POINT('Ctrl Pts',(0.900001215101098,1.14785635641255,0.698771715080855));
#15919=CARTESIAN_POINT('Ctrl Pts',(0.900000537649455,1.14280542295857,0.699580430175527));
#15920=CARTESIAN_POINT('Ctrl Pts',(0.899999997568109,1.13768876957788,0.699999998835552));
#15921=CARTESIAN_POINT('Ctrl Pts',(0.899999999937205,1.13254484130906,0.7));
#15922=CARTESIAN_POINT('Ctrl Pts',(0.9,1.266106713614,0.));
#15923=CARTESIAN_POINT('Ctrl Pts',(0.9,1.26053025554556,0.100869097599589));
#15924=CARTESIAN_POINT('Ctrl Pts',(0.9,1.25495230648558,0.201739398169819));
#15925=CARTESIAN_POINT('Ctrl Pts',(0.9,1.24378819189631,0.403576374532447));
#15926=CARTESIAN_POINT('Ctrl Pts',(0.9,1.23820188085298,0.504545629805417));
#15927=CARTESIAN_POINT('Ctrl Pts',(0.9,1.23261418131727,0.605513513251856));
#15928=CARTESIAN_POINT('Ctrl Pts',(0.900000000000002,-1.266106713614,-8.15320033709099E-17));
#15929=CARTESIAN_POINT('Ctrl Pts',(0.908871090277923,-1.25552568177643,
0.201930159665972));
#15930=CARTESIAN_POINT('Ctrl Pts',(0.917742329685194,-1.24494466498547,
0.403860313587921));
#15931=CARTESIAN_POINT('Ctrl Pts',(0.926613720860141,-1.23436366359623,
0.605790461668883));
#15932=CARTESIAN_POINT('Ctrl Pts',(0.697441255022372,-1.25280938151844,
-5.71013218131409E-5));
#15933=CARTESIAN_POINT('Ctrl Pts',(0.706712389899261,-1.24222855501813,
0.201872952723963));
#15934=CARTESIAN_POINT('Ctrl Pts',(0.71598368260269,-1.23164774534186,0.403803000441224));
#15935=CARTESIAN_POINT('Ctrl Pts',(0.725255135891715,-1.22106695288555,
0.605733041729342));
#15936=CARTESIAN_POINT('Ctrl Pts',(0.494899146035781,-1.23832021354117,
-0.000119230777047918));
#15937=CARTESIAN_POINT('Ctrl Pts',(0.504570354086872,-1.2277396148863,0.201810708652083));
#15938=CARTESIAN_POINT('Ctrl Pts',(0.514241728780064,-1.21715903502506,
0.403740641123913));
#15939=CARTESIAN_POINT('Ctrl Pts',(0.523913273026478,-1.20657847439907,
0.605670566527588));
#15940=CARTESIAN_POINT('Ctrl Pts',(0.292373353339556,-1.22258574808743,
-0.000186633859775947));
#15941=CARTESIAN_POINT('Ctrl Pts',(0.302444661323169,-1.21200540195431,
0.201743181663441));
#15942=CARTESIAN_POINT('Ctrl Pts',(0.312516144861689,-1.20142507679253,
0.403672989556125));
#15943=CARTESIAN_POINT('Ctrl Pts',(0.322587807049886,-1.190844773096,0.605602789690272));
#15944=CARTESIAN_POINT('',(0.32407846024449,-1.19096124572524,0.605603291426262));
#15945=CARTESIAN_POINT('Ctrl Pts',(0.292382661757373,-1.22257596919059,
-1.26634813746307E-16));
#15946=CARTESIAN_POINT('Ctrl Pts',(0.302948004341657,-1.21203750712027,
0.201867748891544));
#15947=CARTESIAN_POINT('Ctrl Pts',(0.313513270922098,-1.20149926476964,
0.403735512620674));
#15948=CARTESIAN_POINT('Ctrl Pts',(0.324078460244491,-1.19096124572524,
0.605603291426262));
#15949=CARTESIAN_POINT('Ctrl Pts',(0.324078460244487,-1.19096124572524,
0.605603291426262));
#15950=CARTESIAN_POINT('Ctrl Pts',(0.515976798438381,-1.20595780001216,
0.605571001180369));
#15951=CARTESIAN_POINT('Ctrl Pts',(0.707956283694857,-1.21982772882273,
0.605541108414459));
#15952=CARTESIAN_POINT('Ctrl Pts',(0.900000000000001,-1.23261418131727,
0.605513513251856));
#15953=CARTESIAN_POINT('Ctrl Pts',(0.906632491847682,-1.13298681949577,
0.7));
#15954=CARTESIAN_POINT('Ctrl Pts',(0.714963137593258,-1.12022681655782,
0.7));
#15955=CARTESIAN_POINT('Ctrl Pts',(0.52336552158394,-1.10638609587519,0.7));
#15956=CARTESIAN_POINT('Ctrl Pts',(0.331856371369197,-1.09142177001972,
0.7));
#15957=CARTESIAN_POINT('Ctrl Pts',(0.904714827274509,-1.16179226195561,
0.7));
#15958=CARTESIAN_POINT('Ctrl Pts',(0.712937153454425,-1.14901967286075,
0.69999980360337));
#15959=CARTESIAN_POINT('Ctrl Pts',(0.521230340369869,-1.13516557394852,
0.700000229443053));
#15960=CARTESIAN_POINT('Ctrl Pts',(0.329608751265076,-1.12018616744754,
0.7));
#15961=CARTESIAN_POINT('Ctrl Pts',(0.901389714107723,-1.21173913866089,
0.676722045797292));
#15962=CARTESIAN_POINT('Ctrl Pts',(0.709425477581998,-1.19894546296063,
0.676731074746188));
#15963=CARTESIAN_POINT('Ctrl Pts',(0.517526696841433,-1.18506766126723,
0.67674067107047));
#15964=CARTESIAN_POINT('Ctrl Pts',(0.325711429829026,-1.17006296935233,
0.676751229163451));
#15965=CARTESIAN_POINT('Ctrl Pts',(0.900079298017777,-1.23142303740181,
0.627132481749528));
#15966=CARTESIAN_POINT('Ctrl Pts',(0.708040181852795,-1.21863106773591,
0.627155851652593));
#15967=CARTESIAN_POINT('Ctrl Pts',(0.516066269599777,-1.20475540724405,
0.627181012790208));
#15968=CARTESIAN_POINT('Ctrl Pts',(0.324172915772929,-1.18975243096407,
0.627208352638976));
#15969=CARTESIAN_POINT('Ctrl Pts',(0.900000000000001,-1.23261418131727,
0.605513513251856));
#15970=CARTESIAN_POINT('Ctrl Pts',(0.707956283694857,-1.21982772882273,
0.605541108414459));
#15971=CARTESIAN_POINT('Ctrl Pts',(0.515976798438381,-1.20595780001216,
0.605571001180369));
#15972=CARTESIAN_POINT('Ctrl Pts',(0.324078460244487,-1.19096124572524,
0.605603291426262));
#15973=CARTESIAN_POINT('',(0.3318563713692,-1.09142177001972,0.7));
#15974=CARTESIAN_POINT('Origin',(0.3318563713692,-1.09142177001972,0.6));
#15975=CARTESIAN_POINT('Ctrl Pts',(0.899999999937167,-1.13254484130906,
0.7));
#15976=CARTESIAN_POINT('Ctrl Pts',(0.710543123935439,-1.11990737114256,
0.7));
#15977=CARTESIAN_POINT('Ctrl Pts',(0.521156529292483,-1.10621348751457,
0.7));
#15978=CARTESIAN_POINT('Ctrl Pts',(0.331856371369197,-1.09142177001972,
0.7));
#15979=CARTESIAN_POINT('Origin',(5.4,-8.11656130105013E-18,0.7));
#15980=CARTESIAN_POINT('',(0.3318563713692,1.09142177001972,0.7));
#15981=CARTESIAN_POINT('',(0.3318563713692,-0.7,0.7));
#15982=CARTESIAN_POINT('Ctrl Pts',(0.3318563713692,1.09142177001972,0.7));
#15983=CARTESIAN_POINT('Ctrl Pts',(0.521156529292483,1.10621348751457,0.7));
#15984=CARTESIAN_POINT('Ctrl Pts',(0.710543123935438,1.11990737114256,0.7));
#15985=CARTESIAN_POINT('Ctrl Pts',(0.899999999937165,1.13254484130906,0.7));
#15986=CARTESIAN_POINT('Ctrl Pts',(0.292373353339556,1.22258574808743,-0.000186633859776018));
#15987=CARTESIAN_POINT('Ctrl Pts',(0.30244466132317,1.21200540195431,0.20174318166344));
#15988=CARTESIAN_POINT('Ctrl Pts',(0.31251614486169,1.20142507679253,0.403672989556124));
#15989=CARTESIAN_POINT('Ctrl Pts',(0.322587807049886,1.190844773096,0.605602789690271));
#15990=CARTESIAN_POINT('Ctrl Pts',(0.494899146035781,1.23832021354117,-0.000119230777047989));
#15991=CARTESIAN_POINT('Ctrl Pts',(0.504570354086872,1.2277396148863,0.201810708652083));
#15992=CARTESIAN_POINT('Ctrl Pts',(0.514241728780064,1.21715903502506,0.403740641123914));
#15993=CARTESIAN_POINT('Ctrl Pts',(0.523913273026478,1.20657847439907,0.605670566527587));
#15994=CARTESIAN_POINT('Ctrl Pts',(0.697441255022371,1.25280938151844,-5.71013218130602E-5));
#15995=CARTESIAN_POINT('Ctrl Pts',(0.70671238989926,1.24222855501813,0.201872952723963));
#15996=CARTESIAN_POINT('Ctrl Pts',(0.715983682602689,1.23164774534186,0.403803000441224));
#15997=CARTESIAN_POINT('Ctrl Pts',(0.725255135891714,1.22106695288555,0.605733041729342));
#15998=CARTESIAN_POINT('Ctrl Pts',(0.9,1.266106713614,1.73472347597681E-18));
#15999=CARTESIAN_POINT('Ctrl Pts',(0.908871090277921,1.25552568177643,0.201930159665973));
#16000=CARTESIAN_POINT('Ctrl Pts',(0.917742329685192,1.24494466498547,0.403860313587921));
#16001=CARTESIAN_POINT('Ctrl Pts',(0.92661372086014,1.23436366359623,0.605790461668883));
#16002=CARTESIAN_POINT('',(0.32407846024449,1.19096124572524,0.605603291426262));
#16003=CARTESIAN_POINT('Ctrl Pts',(0.9,1.23261418131727,0.605513513251856));
#16004=CARTESIAN_POINT('Ctrl Pts',(0.707956283694857,1.21982772882273,0.605541108414459));
#16005=CARTESIAN_POINT('Ctrl Pts',(0.515976798438382,1.20595780001216,0.60557100118037));
#16006=CARTESIAN_POINT('Ctrl Pts',(0.32407846024449,1.19096124572524,0.605603291426262));
#16007=CARTESIAN_POINT('Ctrl Pts',(0.324078460244491,1.19096124572524,0.605603291426262));
#16008=CARTESIAN_POINT('Ctrl Pts',(0.313513270922098,1.20149926476964,0.403735512620674));
#16009=CARTESIAN_POINT('Ctrl Pts',(0.302948004341658,1.21203750712026,0.201867748891544));
#16010=CARTESIAN_POINT('Ctrl Pts',(0.292382661757373,1.22257596919059,3.4477629085039E-17));
#16011=CARTESIAN_POINT('Ctrl Pts',(0.3318563713692,1.09142177001972,0.7));
#16012=CARTESIAN_POINT('Ctrl Pts',(0.523365521583941,1.10638609587519,0.7));
#16013=CARTESIAN_POINT('Ctrl Pts',(0.714963137593258,1.12022681655782,0.7));
#16014=CARTESIAN_POINT('Ctrl Pts',(0.906632491847681,1.13298681949577,0.7));
#16015=CARTESIAN_POINT('Ctrl Pts',(0.329608751265078,1.12018616744754,0.7));
#16016=CARTESIAN_POINT('Ctrl Pts',(0.52123034036987,1.13516557394852,0.700000229443053));
#16017=CARTESIAN_POINT('Ctrl Pts',(0.712937153454426,1.14901967286075,0.699999803603371));
#16018=CARTESIAN_POINT('Ctrl Pts',(0.904714827274509,1.16179226195561,0.700000000000001));
#16019=CARTESIAN_POINT('Ctrl Pts',(0.325711429829028,1.17006296935233,0.676751229163452));
#16020=CARTESIAN_POINT('Ctrl Pts',(0.517526696841433,1.18506766126723,0.67674067107047));
#16021=CARTESIAN_POINT('Ctrl Pts',(0.709425477581997,1.19894546296063,0.676731074746189));
#16022=CARTESIAN_POINT('Ctrl Pts',(0.901389714107722,1.21173913866089,0.676722045797292));
#16023=CARTESIAN_POINT('Ctrl Pts',(0.324172915772932,1.18975243096407,0.627208352638976));
#16024=CARTESIAN_POINT('Ctrl Pts',(0.516066269599778,1.20475540724405,0.627181012790208));
#16025=CARTESIAN_POINT('Ctrl Pts',(0.708040181852794,1.21863106773591,0.627155851652593));
#16026=CARTESIAN_POINT('Ctrl Pts',(0.900079298017776,1.23142303740181,0.627132481749528));
#16027=CARTESIAN_POINT('Ctrl Pts',(0.32407846024449,1.19096124572524,0.605603291426262));
#16028=CARTESIAN_POINT('Ctrl Pts',(0.515976798438382,1.20595780001216,0.60557100118037));
#16029=CARTESIAN_POINT('Ctrl Pts',(0.707956283694857,1.21982772882273,0.605541108414459));
#16030=CARTESIAN_POINT('Ctrl Pts',(0.9,1.23261418131727,0.605513513251856));
#16031=CARTESIAN_POINT('Origin',(0.331856371369202,1.09142177001972,0.6));
#16032=CARTESIAN_POINT('Origin',(0.331856371369202,1.09142177001972,0.6));
#16033=CARTESIAN_POINT('Origin',(0.331856371369201,1.09142177001972,0.6));
#16034=CARTESIAN_POINT('Origin',(0.331856371369202,1.09142177001972,0.6));
#16035=CARTESIAN_POINT('Origin',(10.4681436286308,1.08420482079361,0.6));
#16036=CARTESIAN_POINT('Origin',(10.4681436276939,1.08420482084454,0.6));
#16037=CARTESIAN_POINT('',(10.5680065821063,1.08420482079361,0.605233595624295));
#16038=CARTESIAN_POINT('Origin',(10.4681436286308,1.08420482079361,0.6));
#16039=CARTESIAN_POINT('Origin',(10.4681436286308,1.08420482079361,0.6));
#16040=CARTESIAN_POINT('Origin',(0.3318563713692,-1.09142177001972,0.6));
#16041=CARTESIAN_POINT('Origin',(0.331856371369201,-1.09142177001972,0.6));
#16042=CARTESIAN_POINT('Origin',(0.3318563713692,-1.09142177001972,0.6));
#16043=CARTESIAN_POINT('Origin',(0.3318563713692,-0.7,0.6));
#16044=CARTESIAN_POINT('Ctrl Pts',(0.2922895713475,-1.22266882276207,-0.00177864096060679));
#16045=CARTESIAN_POINT('Ctrl Pts',(0.302885944515497,-1.21209940820877,
0.200681988163859));
#16046=CARTESIAN_POINT('Ctrl Pts',(0.313482241236256,-1.20153021465708,
0.403142632212487));
#16047=CARTESIAN_POINT('Ctrl Pts',(0.324078460244491,-1.19096124572524,
0.605603291426262));
#16048=CARTESIAN_POINT('Ctrl Pts',(0.264022491930188,-1.22039553779506,
-0.000415890128406236));
#16049=CARTESIAN_POINT('Ctrl Pts',(0.274621881512248,-1.20982222712748,
0.202044379074236));
#16050=CARTESIAN_POINT('Ctrl Pts',(0.285221154833576,-1.19924944554801,
0.404504681968985));
#16051=CARTESIAN_POINT('Ctrl Pts',(0.29582042516239,-1.18867654001483,0.606964977361795));
#16052=CARTESIAN_POINT('Ctrl Pts',(0.216712469170969,-1.1940874043406,0.000690255297866666));
#16053=CARTESIAN_POINT('Ctrl Pts',(0.227319688237882,-1.18351239299796,
0.203150045648192));
#16054=CARTESIAN_POINT('Ctrl Pts',(0.237926932441998,-1.17293746916702,
0.405609838636422));
#16055=CARTESIAN_POINT('Ctrl Pts',(0.248534117816369,-1.1623628476683,0.608069650238703));
#16056=CARTESIAN_POINT('Ctrl Pts',(0.200219987929043,-1.14439035743082,
-0.00103956457010847));
#16057=CARTESIAN_POINT('Ctrl Pts',(0.210830491339948,-1.13382006821851,
0.201420337884579));
#16058=CARTESIAN_POINT('Ctrl Pts',(0.221440906577676,-1.12324995278282,
0.403880253819325));
#16059=CARTESIAN_POINT('Ctrl Pts',(0.232051411471599,-1.11268010558856,
0.606340179010355));
#16060=CARTESIAN_POINT('Ctrl Pts',(0.200161975173303,-1.12312592850316,
-0.00214651389202307));
#16061=CARTESIAN_POINT('Ctrl Pts',(0.210772455448684,-1.11255764422181,
0.200313510564959));
#16062=CARTESIAN_POINT('Ctrl Pts',(0.221382936352032,-1.1019895901204,0.402773547004277));
#16063=CARTESIAN_POINT('Ctrl Pts',(0.231993417893744,-1.09142177001972,
0.605233595624295));
#16064=CARTESIAN_POINT('Origin',(10.4681436286308,-1.08420482109828,0.6));
#16065=CARTESIAN_POINT('',(10.5680065821063,-1.08420482079361,0.605233595624295));
#16066=CARTESIAN_POINT('Origin',(10.4681436286308,-1.08420482099672,0.600000000000001));
#16067=CARTESIAN_POINT('Origin',(10.4681436286308,-1.08420482109828,0.6));
#16068=CARTESIAN_POINT('Origin',(10.4681436286308,0.7,0.6));
#16069=CARTESIAN_POINT('',(10.5680065821063,0.7,0.605233595624295));
#16070=CARTESIAN_POINT('Ctrl Pts',(10.599839982685,-1.11594741464673,-0.00218387205330164));
#16071=CARTESIAN_POINT('Ctrl Pts',(10.5892288496247,-1.10536637943871,0.200288608282177));
#16072=CARTESIAN_POINT('Ctrl Pts',(10.5786177161011,-1.0947855138519,0.402761097457634));
#16073=CARTESIAN_POINT('Ctrl Pts',(10.5680065821063,-1.08420482079362,0.605233595624295));
#16074=CARTESIAN_POINT('Ctrl Pts',(10.5997613205547,-1.14474784499259,-0.000682909193257743));
#16075=CARTESIAN_POINT('Ctrl Pts',(10.5891501209488,-1.13416481604349,0.201789447273867));
#16076=CARTESIAN_POINT('Ctrl Pts',(10.5785391399155,-1.12358205581644,0.404261829287571));
#16077=CARTESIAN_POINT('Ctrl Pts',(10.5679279386544,-1.11299934606825,0.606734202078189));
#16078=CARTESIAN_POINT('Ctrl Pts',(10.5764119435127,-1.19466846760808,0.000702210001053139));
#16079=CARTESIAN_POINT('Ctrl Pts',(10.5658041809617,-1.18408222297768,0.203174550667819));
#16080=CARTESIAN_POINT('Ctrl Pts',(10.5551963844732,-1.17349608774572,0.405646894856767));
#16081=CARTESIAN_POINT('Ctrl Pts',(10.544588659013,-1.16291012508165,0.608119251464957));
#16082=CARTESIAN_POINT('Ctrl Pts',(10.5269342003857,-1.21442651155969,-0.000858270497959616));
#16083=CARTESIAN_POINT('Ctrl Pts',(10.5163317654776,-1.20384274018949,0.201614467507756));
#16084=CARTESIAN_POINT('Ctrl Pts',(10.5057293269973,-1.1932591813998,0.404087216090532));
#16085=CARTESIAN_POINT('Ctrl Pts',(10.4951269905998,-1.18267571840064,0.606559974437339));
#16086=CARTESIAN_POINT('Ctrl Pts',(10.5053655128635,-1.21565094114741,-0.0019246498908503));
#16087=CARTESIAN_POINT('Ctrl Pts',(10.4947646468921,-1.20506932615592,0.200548282383137));
#16088=CARTESIAN_POINT('Ctrl Pts',(10.4841638390504,-1.19448787589602,0.403021225840181));
#16089=CARTESIAN_POINT('Ctrl Pts',(10.4735630903435,-1.18390659316268,0.605494180667945));
#16090=CARTESIAN_POINT('Ctrl Pts',(10.5997255308004,-1.11583328740478,1.02782365951626E-16));
#16091=CARTESIAN_POINT('Ctrl Pts',(10.589152548365,-1.10529029582828,0.201744523047832));
#16092=CARTESIAN_POINT('Ctrl Pts',(10.5785795654695,-1.09474747266587,0.40348905487273));
#16093=CARTESIAN_POINT('Ctrl Pts',(10.5680065821063,-1.08420482079362,0.605233595624295));
#16094=CARTESIAN_POINT('Ctrl Pts',(10.5053638082297,1.21564923960921,-0.0018920919656423));
#16095=CARTESIAN_POINT('Ctrl Pts',(10.4947635104759,1.20506819181477,0.200569987667808));
#16096=CARTESIAN_POINT('Ctrl Pts',(10.4841632708454,1.19448730873444,0.403032078483127));
#16097=CARTESIAN_POINT('Ctrl Pts',(10.4735630903435,1.18390659316268,0.605494180667945));
#16098=CARTESIAN_POINT('Ctrl Pts',(10.5341220579192,1.21401666636749,-0.000470252816738081));
#16099=CARTESIAN_POINT('Ctrl Pts',(10.5235196325477,1.20343268662274,0.201991562854702));
#16100=CARTESIAN_POINT('Ctrl Pts',(10.5129172908767,1.19284910679518,0.404453403808947));
#16101=CARTESIAN_POINT('Ctrl Pts',(10.5023149573519,1.18226542681329,0.606915239027137));
#16102=CARTESIAN_POINT('Ctrl Pts',(10.5827170203615,1.18801090922716,0.000717463067903341));
#16103=CARTESIAN_POINT('Ctrl Pts',(10.5721088691741,1.17742555398174,0.203178921531494));
#16104=CARTESIAN_POINT('Ctrl Pts',(10.5615007184277,1.16684027916303,0.405640383775807));
#16105=CARTESIAN_POINT('Ctrl Pts',(10.5508925935528,1.15625520969485,0.60810185787831));
#16106=CARTESIAN_POINT('Ctrl Pts',(10.5997792798033,1.13754603572512,-0.00102559206997387));
#16107=CARTESIAN_POINT('Ctrl Pts',(10.5891686973038,1.12696411138589,0.201435946515793));
#16108=CARTESIAN_POINT('Ctrl Pts',(10.5785581831385,1.11638231376635,0.40389749513889));
#16109=CARTESIAN_POINT('Ctrl Pts',(10.5679475995174,1.10580071474959,0.606359050464716));
#16110=CARTESIAN_POINT('Ctrl Pts',(10.5998382764002,1.11594571320176,-0.00215131420076595));
#16111=CARTESIAN_POINT('Ctrl Pts',(10.5892277121014,1.10536524516024,0.200310313518148));
#16112=CARTESIAN_POINT('Ctrl Pts',(10.5786171473394,1.09478494672192,0.402771950076102));
#16113=CARTESIAN_POINT('Ctrl Pts',(10.5680065821063,1.08420482079361,0.605233595624295));
#16114=CARTESIAN_POINT('Ctrl Pts',(10.5680065821063,1.08420482079361,0.605233595624295));
#16115=CARTESIAN_POINT('Ctrl Pts',(10.5785795654695,1.09474747266587,0.40348905487273));
#16116=CARTESIAN_POINT('Ctrl Pts',(10.589152548365,1.10529029582828,0.201744523047831));
#16117=CARTESIAN_POINT('Ctrl Pts',(10.5997255308004,1.11583328740478,1.07661275727811E-16));
#16118=CARTESIAN_POINT('Ctrl Pts',(10.1947388861048,1.09885088260187,0.7));
#16119=CARTESIAN_POINT('Ctrl Pts',(10.285877616441,1.09404209584202,0.7));
#16120=CARTESIAN_POINT('Ctrl Pts',(10.3770124662346,1.0891584122264,0.7));
#16121=CARTESIAN_POINT('Ctrl Pts',(10.4681436286308,1.08420482079361,0.7));
#16122=CARTESIAN_POINT('Ctrl Pts',(10.196260416419,1.12768774893097,0.700000000000001));
#16123=CARTESIAN_POINT('Ctrl Pts',(10.2874149314686,1.12287675076168,0.699999949550842));
#16124=CARTESIAN_POINT('Ctrl Pts',(10.3785648662465,1.11799094453753,0.700000051218742));
#16125=CARTESIAN_POINT('Ctrl Pts',(10.4697107510168,1.11303515260326,0.7));
#16126=CARTESIAN_POINT('Ctrl Pts',(10.1988975981852,1.17766904563614,0.67669140632491));
#16127=CARTESIAN_POINT('Ctrl Pts',(10.2900793016129,1.17285439035486,0.676693724638983));
#16128=CARTESIAN_POINT('Ctrl Pts',(10.3812557252598,1.16796482352885,0.676696026813929));
#16129=CARTESIAN_POINT('Ctrl Pts',(10.4724269697127,1.16300539549315,0.676698381019544));
#16130=CARTESIAN_POINT('Ctrl Pts',(10.1999375452555,1.19737868557977,0.627098033786781));
#16131=CARTESIAN_POINT('Ctrl Pts',(10.2911301919381,1.19256517083271,0.627104033151799));
#16132=CARTESIAN_POINT('Ctrl Pts',(10.382317043787,1.18767684023183,0.627110048826767));
#16133=CARTESIAN_POINT('Ctrl Pts',(10.4734985149421,1.18271860027509,0.627116141711795));
#16134=CARTESIAN_POINT('Ctrl Pts',(10.1999999975038,1.19856231440453,0.605472757505366));
#16135=CARTESIAN_POINT('Ctrl Pts',(10.2911933328565,1.19375025772558,0.605479840815741));
#16136=CARTESIAN_POINT('Ctrl Pts',(10.3823809652617,1.18886335120032,0.605486986548286));
#16137=CARTESIAN_POINT('Ctrl Pts',(10.4735630903435,1.18390659316268,0.605494180667944));
#16138=CARTESIAN_POINT('Ctrl Pts',(0.200159601751749,1.12312829248604,-0.00219180147311912));
#16139=CARTESIAN_POINT('Ctrl Pts',(0.210770873167554,1.11255922017607,0.200283318842441));
#16140=CARTESIAN_POINT('Ctrl Pts',(0.221382145211419,1.10199037808008,0.402758451142111));
#16141=CARTESIAN_POINT('Ctrl Pts',(0.231993417893744,1.09142177001972,0.605233595624295));
#16142=CARTESIAN_POINT('Ctrl Pts',(0.200236952094631,1.15148086499205,-0.000715869007730825));
#16143=CARTESIAN_POINT('Ctrl Pts',(0.210848310847714,1.14090905181173,0.201759082033021));
#16144=CARTESIAN_POINT('Ctrl Pts',(0.221459381762758,1.13033759660317,0.404234066901971));
#16145=CARTESIAN_POINT('Ctrl Pts',(0.232070742664217,1.11976621744484,0.606709040139042));
#16146=CARTESIAN_POINT('Ctrl Pts',(0.222806696702742,1.20067708175657,0.000669311976984441));
#16147=CARTESIAN_POINT('Ctrl Pts',(0.233413416075889,1.19010082554658,0.203144236955742));
#16148=CARTESIAN_POINT('Ctrl Pts',(0.244020198555212,1.17952469009474,0.405619164345205));
#16149=CARTESIAN_POINT('Ctrl Pts',(0.254626870458834,1.16894881850735,0.608094110943904));
#16150=CARTESIAN_POINT('Ctrl Pts',(0.271086891015657,1.22096622390789,-0.000801865493577694));
#16151=CARTESIAN_POINT('Ctrl Pts',(0.281686280594249,1.21039315447922,0.201673594461172));
#16152=CARTESIAN_POINT('Ctrl Pts',(0.292285672737775,1.1998203699977,0.404149068703718));
#16153=CARTESIAN_POINT('Ctrl Pts',(0.302884933932915,1.18924771644243,0.606624555877912));
#16154=CARTESIAN_POINT('Ctrl Pts',(0.292287201081515,1.22267118699778,-0.00182392867695869));
#16155=CARTESIAN_POINT('Ctrl Pts',(0.302884364349574,1.21210098433295,0.200651796350731));
#16156=CARTESIAN_POINT('Ctrl Pts',(0.313481451159089,1.20153100270242,0.403127536304793));
#16157=CARTESIAN_POINT('Ctrl Pts',(0.324078460244491,1.19096124572524,0.605603291426262));
#16158=CARTESIAN_POINT('Origin',(10.6002740930491,1.4,-0.0104671912485891));
#16159=CARTESIAN_POINT('Origin',(0.331856371369202,1.09142177001972,0.6));
#16160=CARTESIAN_POINT('',(0.3318563713692,1.09142177001972,0.9));
#16161=CARTESIAN_POINT('',(0.0322675109428288,1.09142177001972,0.615700786872883));
#16162=CARTESIAN_POINT('Origin',(0.3318563713692,1.09142177001972,0.6));
#16163=CARTESIAN_POINT('',(0.308522637995069,1.39004019713626,0.616809874278785));
#16164=CARTESIAN_POINT('Origin',(0.331856371369202,1.09142177001972,0.6));
#16165=CARTESIAN_POINT('Origin',(0.331856371369201,1.09142177001972,0.6));
#16166=CARTESIAN_POINT('Origin',(10.4681436286308,1.08420482079361,0.6));
#16167=CARTESIAN_POINT('',(10.4681436286308,1.08420482109828,0.9));
#16168=CARTESIAN_POINT('',(10.4844020137689,1.3833101379008,0.616482542003833));
#16169=CARTESIAN_POINT('Origin',(10.4681436258201,1.08420482094639,0.6));
#16170=CARTESIAN_POINT('',(10.7677324890572,1.08420482079361,0.615700786872884));
#16171=CARTESIAN_POINT('Origin',(10.4681436286308,1.08420482079361,0.6));
#16172=CARTESIAN_POINT('Origin',(10.4681436286308,1.08420482079362,0.6));
#16173=CARTESIAN_POINT('Origin',(0.3318563713692,-1.09142177001972,0.6));
#16174=CARTESIAN_POINT('',(0.3318563713692,-1.09142177001972,0.9));
#16175=CARTESIAN_POINT('',(0.308522637995069,-1.39004019713626,0.616809874278785));
#16176=CARTESIAN_POINT('Origin',(0.3318563713692,-1.09142177001972,0.6));
#16177=CARTESIAN_POINT('',(0.0322675109428289,-1.09142177001972,0.615700786872884));
#16178=CARTESIAN_POINT('Origin',(0.3318563713692,-1.09142177001972,0.6));
#16179=CARTESIAN_POINT('Origin',(0.331856371369201,-1.09142177001972,0.6));
#16180=CARTESIAN_POINT('Origin',(0.3318563713692,-0.7,0.6));
#16181=CARTESIAN_POINT('',(0.0322675109428288,-0.7,0.615700786872883));
#16182=CARTESIAN_POINT('',(0.3318563713692,-0.7,0.9));
#16183=CARTESIAN_POINT('Ctrl Pts',(0.276048389810261,-1.42252533450788,
-0.00533608639730399));
#16184=CARTESIAN_POINT('Ctrl Pts',(0.28687338241706,-1.4116967417008,0.202045878554724));
#16185=CARTESIAN_POINT('Ctrl Pts',(0.297698133178874,-1.40086836142621,
0.409427865329919));
#16186=CARTESIAN_POINT('Ctrl Pts',(0.308522637995069,-1.39004019713626,
0.616809874278785));
#16187=CARTESIAN_POINT('Ctrl Pts',(0.191246496057484,-1.41570630783033,
-0.00124775669238285));
#16188=CARTESIAN_POINT('Ctrl Pts',(0.202080757839133,-1.40486573978029,
0.206133102090467));
#16189=CARTESIAN_POINT('Ctrl Pts',(0.212914648880055,-1.39402634701096,
0.413514041581016));
#16190=CARTESIAN_POINT('Ctrl Pts',(0.223748532748767,-1.38318608000504,
0.620894932085382));
#16191=CARTESIAN_POINT('Ctrl Pts',(0.0492682973509243,-1.33685850703924,
0.00207719607616587));
#16192=CARTESIAN_POINT('Ctrl Pts',(0.0601266125734448,-1.32601270457081,
0.209456583216085));
#16193=CARTESIAN_POINT('Ctrl Pts',(0.0709850253737815,-1.3151666447344,
0.416835949794532));
#16194=CARTESIAN_POINT('Ctrl Pts',(0.0818432319483421,-1.30432109509162,
0.624215353109623));
#16195=CARTESIAN_POINT('Ctrl Pts',(-0.000163444061205068,-1.18769013309795,
-0.00311869847265479));
#16196=CARTESIAN_POINT('Ctrl Pts',(0.0107049555364969,-1.17685886333949,
0.204261034729081));
#16197=CARTESIAN_POINT('Ctrl Pts',(0.0215730900970294,-1.16602762920277,
0.411640782964944));
#16198=CARTESIAN_POINT('Ctrl Pts',(0.0324414916763936,-1.15519677672624,
0.619020537031064));
#16199=CARTESIAN_POINT('Ctrl Pts',(-0.00033748371827097,-1.12389640457412,
-0.0064395729582146));
#16200=CARTESIAN_POINT('Ctrl Pts',(0.0105308471731094,-1.11307128361434,
0.200940534347673));
#16201=CARTESIAN_POINT('Ctrl Pts',(0.0213991787230862,-1.10224640406117,
0.408320654220332));
#16202=CARTESIAN_POINT('Ctrl Pts',(0.0322675109428289,-1.09142177001972,
0.615700786872884));
#16203=CARTESIAN_POINT('Ctrl Pts',(0.27632692456468,-1.42224670711126,5.13911829758129E-17));
#16204=CARTESIAN_POINT('Ctrl Pts',(0.287059068122268,-1.41151099373342,
0.20560326985903));
#16205=CARTESIAN_POINT('Ctrl Pts',(0.297790973931072,-1.40077548928706,
0.411206561171438));
#16206=CARTESIAN_POINT('Ctrl Pts',(0.308522637995069,-1.39004019713626,
0.616809874278785));
#16207=CARTESIAN_POINT('Ctrl Pts',(0.0322675109428289,-1.09142177001972,
0.615700786872884));
#16208=CARTESIAN_POINT('Ctrl Pts',(0.0215116733095221,-1.10213436178043,
0.410467178800746));
#16209=CARTESIAN_POINT('Ctrl Pts',(0.0107558363321879,-1.11284719399673,
0.205233583245308));
#16210=CARTESIAN_POINT('Ctrl Pts',(1.76901136968166E-16,-1.12356026268968,
-7.45931094670027E-17));
#16211=CARTESIAN_POINT('Origin',(10.4681436286308,-1.08420482109828,0.6));
#16212=CARTESIAN_POINT('',(10.7677324890572,-1.08420482079361,0.615700786872884));
#16213=CARTESIAN_POINT('',(10.4844020137689,-1.3833101379008,0.616482542003833));
#16214=CARTESIAN_POINT('Origin',(10.4681436286308,-1.08420482079361,0.600000000000001));
#16215=CARTESIAN_POINT('',(10.4681436258201,-1.08420482094639,0.9));
#16216=CARTESIAN_POINT('Origin',(10.4681436286308,-1.08420482109828,0.6));
#16217=CARTESIAN_POINT('Origin',(10.4681436286308,-1.08420482079361,0.6));
#16218=CARTESIAN_POINT('Origin',(10.4681436286308,0.7,0.6));
#16219=CARTESIAN_POINT('',(10.7677324890572,0.7,0.615700786872884));
#16220=CARTESIAN_POINT('',(10.4681436286308,0.7,0.9));
#16221=CARTESIAN_POINT('Ctrl Pts',(10.4681436286308,-1.08420482079361,0.9));
#16222=CARTESIAN_POINT('Ctrl Pts',(9.02115959826777,-1.16285813221549,0.9));
#16223=CARTESIAN_POINT('Ctrl Pts',(5.64262097844114,-1.30550334054488,0.9));
#16224=CARTESIAN_POINT('Ctrl Pts',(2.25816172369615,-1.24194126716656,0.9));
#16225=CARTESIAN_POINT('Ctrl Pts',(0.331856371369198,-1.09142177001972,
0.9));
#16226=CARTESIAN_POINT('Ctrl Pts',(10.4728449957889,-1.17069581622255,0.9));
#16227=CARTESIAN_POINT('Ctrl Pts',(9.02515960257209,-1.24945398332951,0.900002463983243));
#16228=CARTESIAN_POINT('Ctrl Pts',(5.64406008560805,-1.39235654229312,0.899995181674544));
#16229=CARTESIAN_POINT('Ctrl Pts',(2.25481214769604,-1.3286896492945,0.900006992415263));
#16230=CARTESIAN_POINT('Ctrl Pts',(0.325113511056834,-1.17771496230318,
0.9));
#16231=CARTESIAN_POINT('Ctrl Pts',(10.4809942371438,-1.32061731204901,0.830050158657121));
#16232=CARTESIAN_POINT('Ctrl Pts',(9.03210079995546,-1.3995487214628,0.829938185878055));
#16233=CARTESIAN_POINT('Ctrl Pts',(5.64656962219688,-1.54290142969263,0.82970437227026));
#16234=CARTESIAN_POINT('Ctrl Pts',(2.24896854757963,-1.47903552984056,0.829838703712927));
#16235=CARTESIAN_POINT('Ctrl Pts',(0.313425270489114,-1.32729771265557,
0.830156825336737));
#16236=CARTESIAN_POINT('Ctrl Pts',(10.4842082875648,-1.37974615923803,0.681348425135383));
#16237=CARTESIAN_POINT('Ctrl Pts',(9.03482793853036,-1.45862084618981,0.681058092399338));
#16238=CARTESIAN_POINT('Ctrl Pts',(5.64753778607331,-1.60187726023264,0.68045297450285));
#16239=CARTESIAN_POINT('Ctrl Pts',(2.24670449952385,-1.53809938127555,0.680799765935021));
#16240=CARTESIAN_POINT('Ctrl Pts',(0.308806004580392,-1.38641375285276,
0.681625057916928));
#16241=CARTESIAN_POINT('Ctrl Pts',(10.4844020137689,-1.3833101379008,0.616482542003833));
#16242=CARTESIAN_POINT('Ctrl Pts',(9.03499042108131,-1.46211428773623,0.616139856494792));
#16243=CARTESIAN_POINT('Ctrl Pts',(5.64759185703765,-1.60522711936681,0.615422163720642));
#16244=CARTESIAN_POINT('Ctrl Pts',(2.24657199659733,-1.54153220865049,0.615835494619844));
#16245=CARTESIAN_POINT('Ctrl Pts',(0.308522637995066,-1.39004019713626,
0.616809874278785));
#16246=CARTESIAN_POINT('Ctrl Pts',(0.308522637995066,-1.39004019713626,
0.616809874278785));
#16247=CARTESIAN_POINT('Ctrl Pts',(2.24657199659733,-1.54153220865049,0.615835494619844));
#16248=CARTESIAN_POINT('Ctrl Pts',(5.64759185703765,-1.60522711936681,0.615422163720642));
#16249=CARTESIAN_POINT('Ctrl Pts',(9.03499042108131,-1.46211428773623,0.616139856494792));
#16250=CARTESIAN_POINT('Ctrl Pts',(10.4844020137689,-1.3833101379008,0.616482542003833));
#16251=CARTESIAN_POINT('Ctrl Pts',(10.4681436258201,-1.08420482094639,0.900000000000001));
#16252=CARTESIAN_POINT('Ctrl Pts',(9.02115959639274,-1.16285813229465,0.9));
#16253=CARTESIAN_POINT('Ctrl Pts',(5.64262097750198,-1.30550334052724,0.9));
#16254=CARTESIAN_POINT('Ctrl Pts',(2.25816172369615,-1.24194126716656,0.9));
#16255=CARTESIAN_POINT('Ctrl Pts',(0.331856371369198,-1.09142177001972,
0.9));
#16256=CARTESIAN_POINT('Ctrl Pts',(10.8003433549902,-1.11672267507076,-0.00655160349952438));
#16257=CARTESIAN_POINT('Ctrl Pts',(10.7894730668347,-1.10588321133639,0.200865850630566));
#16258=CARTESIAN_POINT('Ctrl Pts',(10.7786027781932,-1.09504392553578,0.408283314033857));
#16259=CARTESIAN_POINT('Ctrl Pts',(10.7677324890572,-1.08420482079361,0.615700786872885));
#16260=CARTESIAN_POINT('Ctrl Pts',(10.8001073672393,-1.20312439623403,-0.00204868896805508));
#16261=CARTESIAN_POINT('Ctrl Pts',(10.7892368724076,-1.19227880391739,0.205368384315645));
#16262=CARTESIAN_POINT('Ctrl Pts',(10.7783670568079,-1.18143370221047,0.41278551899075));
#16263=CARTESIAN_POINT('Ctrl Pts',(10.7674965587017,-1.17058839661753,0.620202606234566));
#16264=CARTESIAN_POINT('Ctrl Pts',(10.7300137544668,-1.35289768637741,0.00210488808650419));
#16265=CARTESIAN_POINT('Ctrl Pts',(10.7191538066016,-1.34204221082848,0.209521911971666));
#16266=CARTESIAN_POINT('Ctrl Pts',(10.7082938463195,-1.33118673671862,0.416938933985702));
#16267=CARTESIAN_POINT('Ctrl Pts',(10.6974340169938,-1.32033143065575,0.624355970618915));
#16268=CARTESIAN_POINT('Ctrl Pts',(10.5816241002662,-1.4121605627967,-0.00257485550010117));
#16269=CARTESIAN_POINT('Ctrl Pts',(10.5707805459565,-1.4013126969686,0.204843391064434));
#16270=CARTESIAN_POINT('Ctrl Pts',(10.5599369567012,-1.39046512672587,0.412261650129749));
#16271=CARTESIAN_POINT('Ctrl Pts',(10.5490937145378,-1.37961751361469,0.619679923312015));
#16272=CARTESIAN_POINT('Ctrl Pts',(10.5169176890673,-1.41583338198674,-0.00577403633861717));
#16273=CARTESIAN_POINT('Ctrl Pts',(10.5060789456421,-1.40499213715574,0.201644806368331));
#16274=CARTESIAN_POINT('Ctrl Pts',(10.4952403861233,-1.39415105487295,0.40906366572247));
#16275=CARTESIAN_POINT('Ctrl Pts',(10.4844020137689,-1.3833101379008,0.616482542003833));
#16276=CARTESIAN_POINT('Ctrl Pts',(10.8,-1.11638029377732,-2.51534904016637E-17));
#16277=CARTESIAN_POINT('Ctrl Pts',(10.7892441634977,-1.10565496086826,0.205233586491178));
#16278=CARTESIAN_POINT('Ctrl Pts',(10.7784883265195,-1.09492980219801,0.410467182062988));
#16279=CARTESIAN_POINT('Ctrl Pts',(10.7677324890572,-1.08420482079361,0.615700786872885));
#16280=CARTESIAN_POINT('Ctrl Pts',(10.4844020137689,-1.3833101379008,0.616482542003833));
#16281=CARTESIAN_POINT('Ctrl Pts',(10.4951398148107,-1.39405045994841,0.410988344812119));
#16282=CARTESIAN_POINT('Ctrl Pts',(10.5058777995597,-1.40479094425298,0.205494164234945));
#16283=CARTESIAN_POINT('Ctrl Pts',(10.5166159648474,-1.4155315881283,-2.5652223401007E-16));
#16284=CARTESIAN_POINT('Ctrl Pts',(10.5169125872774,1.41582827901939,-0.0056764044152427));
#16285=CARTESIAN_POINT('Ctrl Pts',(10.5060755445066,1.40498873522851,0.20170989432247));
#16286=CARTESIAN_POINT('Ctrl Pts',(10.4952386855848,1.39414935393528,0.409096209702196));
#16287=CARTESIAN_POINT('Ctrl Pts',(10.4844020137689,1.3833101379008,0.616482542003833));
#16288=CARTESIAN_POINT('Ctrl Pts',(10.6031877991504,1.41093118264609,-0.00141083033817288));
#16289=CARTESIAN_POINT('Ctrl Pts',(10.5923442181457,1.40008262840665,0.205974657203891));
#16290=CARTESIAN_POINT('Ctrl Pts',(10.5815009048179,1.38923496752292,0.413360205434192));
#16291=CARTESIAN_POINT('Ctrl Pts',(10.5706576147941,1.37838663885266,0.62074571708141));
#16292=CARTESIAN_POINT('Ctrl Pts',(10.7489822201969,1.33286898269122,0.00215046584238339));
#16293=CARTESIAN_POINT('Ctrl Pts',(10.7381210493968,1.32201618867047,0.209534855263179));
#16294=CARTESIAN_POINT('Ctrl Pts',(10.7272598662103,1.31116338896628,0.416919242515175));
#16295=CARTESIAN_POINT('Ctrl Pts',(10.716398780155,1.30031077634578,0.624303643734563));
#16296=CARTESIAN_POINT('Ctrl Pts',(10.8001612475457,1.18151886169146,-0.00307678645922502));
#16297=CARTESIAN_POINT('Ctrl Pts',(10.7892926103682,1.17067663552019,0.20430785074418));
#16298=CARTESIAN_POINT('Ctrl Pts',(10.7784241800195,1.15983442267521,0.41169249890798));
#16299=CARTESIAN_POINT('Ctrl Pts',(10.7675555412906,1.14899250266155,0.619077151394146));
#16300=CARTESIAN_POINT('Ctrl Pts',(10.8003382383521,1.11671757294177,-0.00645397222975308));
#16301=CARTESIAN_POINT('Ctrl Pts',(10.7894696557425,1.1058798099729,0.200930938146656));
#16302=CARTESIAN_POINT('Ctrl Pts',(10.778601072647,1.09504222488243,0.408315857793383));
#16303=CARTESIAN_POINT('Ctrl Pts',(10.7677324890572,1.08420482079361,0.615700786872884));
#16304=CARTESIAN_POINT('Ctrl Pts',(10.5166159648474,1.4155315881283,3.37837396946483E-16));
#16305=CARTESIAN_POINT('Ctrl Pts',(10.5058777995597,1.40479094425298,0.205494164234944));
#16306=CARTESIAN_POINT('Ctrl Pts',(10.4951398148107,1.39405045994841,0.41098834481212));
#16307=CARTESIAN_POINT('Ctrl Pts',(10.4844020137689,1.3833101379008,0.616482542003833));
#16308=CARTESIAN_POINT('Ctrl Pts',(10.7677324890572,1.08420482079361,0.615700786872884));
#16309=CARTESIAN_POINT('Ctrl Pts',(10.7784883265195,1.09492980219801,0.410467182062988));
#16310=CARTESIAN_POINT('Ctrl Pts',(10.7892441634977,1.10565496086826,0.205233586491177));
#16311=CARTESIAN_POINT('Ctrl Pts',(10.8,1.11638029377732,-4.7271214720368E-17));
#16312=CARTESIAN_POINT('Ctrl Pts',(0.3318563713692,1.09142177001972,0.9));
#16313=CARTESIAN_POINT('Ctrl Pts',(1.77658538561441,1.20431139287985,0.9));
#16314=CARTESIAN_POINT('Ctrl Pts',(5.15852145577913,1.31798734362749,0.900000000000001));
#16315=CARTESIAN_POINT('Ctrl Pts',(8.53883158814675,1.18907590268945,0.9));
#16316=CARTESIAN_POINT('Ctrl Pts',(10.4681436286308,1.08420482079361,0.9));
#16317=CARTESIAN_POINT('Ctrl Pts',(0.325113511056836,1.17771496230318,0.9));
#16318=CARTESIAN_POINT('Ctrl Pts',(1.77238748853623,1.29094597754667,0.900005244311447));
#16319=CARTESIAN_POINT('Ctrl Pts',(5.15940689953628,1.40489117512763,0.899995532233175));
#16320=CARTESIAN_POINT('Ctrl Pts',(8.54259780483314,1.2757067056985,0.90000328531099));
#16321=CARTESIAN_POINT('Ctrl Pts',(10.4728449957889,1.17069581622255,0.9));
#16322=CARTESIAN_POINT('Ctrl Pts',(0.313425270489116,1.32729771265557,0.830156825336737));
#16323=CARTESIAN_POINT('Ctrl Pts',(1.76508272830699,1.44110107554431,0.829918234118879));
#16324=CARTESIAN_POINT('Ctrl Pts',(5.16095094050242,1.55552201031752,0.829677185710002));
#16325=CARTESIAN_POINT('Ctrl Pts',(8.54913632089268,1.4258591912674,0.829900861618366));
#16326=CARTESIAN_POINT('Ctrl Pts',(10.4809942371438,1.32061731204901,0.830050158657121));
#16327=CARTESIAN_POINT('Ctrl Pts',(0.308806004580394,1.38641375285276,0.681625057916928));
#16328=CARTESIAN_POINT('Ctrl Pts',(1.76222987578798,1.50017797416985,0.681006088930498));
#16329=CARTESIAN_POINT('Ctrl Pts',(5.16154986224672,1.61450132085358,0.68038246417749));
#16330=CARTESIAN_POINT('Ctrl Pts',(8.55170115551887,1.48491240850707,0.680961314820656));
#16331=CARTESIAN_POINT('Ctrl Pts',(10.4842082875648,1.37974615923803,0.681348425135383));
#16332=CARTESIAN_POINT('Ctrl Pts',(0.308522637995068,1.39004019713626,0.616809874278785));
#16333=CARTESIAN_POINT('Ctrl Pts',(1.76205965694675,1.50365920577193,0.616079089534579));
#16334=CARTESIAN_POINT('Ctrl Pts',(5.16158497046229,1.61783515152865,0.615338844765104));
#16335=CARTESIAN_POINT('Ctrl Pts',(8.55185322351876,1.48838233768137,0.616025627991778));
#16336=CARTESIAN_POINT('Ctrl Pts',(10.4844020137689,1.3833101379008,0.616482542003833));
#16337=CARTESIAN_POINT('Ctrl Pts',(10.4844020137689,1.3833101379008,0.616482542003833));
#16338=CARTESIAN_POINT('Ctrl Pts',(8.55185322351876,1.48838233768137,0.616025627991778));
#16339=CARTESIAN_POINT('Ctrl Pts',(5.16158497046229,1.61783515152865,0.615338844765104));
#16340=CARTESIAN_POINT('Ctrl Pts',(1.76205965694675,1.50365920577193,0.616079089534579));
#16341=CARTESIAN_POINT('Ctrl Pts',(0.308522637995068,1.39004019713626,0.616809874278785));
#16342=CARTESIAN_POINT('Ctrl Pts',(0.3318563713692,1.09142177001972,0.9));
#16343=CARTESIAN_POINT('Ctrl Pts',(1.77658538561441,1.20431139287985,0.9));
#16344=CARTESIAN_POINT('Ctrl Pts',(5.15852145577913,1.31798734362749,0.900000000000001));
#16345=CARTESIAN_POINT('Ctrl Pts',(8.53883158814675,1.18907590268945,0.9));
#16346=CARTESIAN_POINT('Ctrl Pts',(10.4681436286308,1.08420482079361,0.9));
#16347=CARTESIAN_POINT('Ctrl Pts',(-0.000344602063817145,1.12390349461883,
-0.00657539908256866));
#16348=CARTESIAN_POINT('Ctrl Pts',(0.0105261016091243,1.11307601020539,
0.200849983592616));
#16349=CARTESIAN_POINT('Ctrl Pts',(0.0213968059409475,1.10224876730309,
0.408275378840013));
#16350=CARTESIAN_POINT('Ctrl Pts',(0.0322675109428289,1.09142177001972,
0.615700786872884));
#16351=CARTESIAN_POINT('Ctrl Pts',(-0.000112549170678945,1.2089618047365,
-0.00214756610981592));
#16352=CARTESIAN_POINT('Ctrl Pts',(0.0107584275574203,1.19812589474889,
0.205277296000037));
#16353=CARTESIAN_POINT('Ctrl Pts',(0.021628504370896,1.18729063034778,0.412702239156743));
#16354=CARTESIAN_POINT('Ctrl Pts',(0.0324994852542487,1.17645511229507,
0.620127120417125));
#16355=CARTESIAN_POINT('Ctrl Pts',(0.0675181008536004,1.35659180908255,
0.00201426213057289));
#16356=CARTESIAN_POINT('Ctrl Pts',(0.0783748317004002,1.34574224493831,
0.20943904356877));
#16357=CARTESIAN_POINT('Ctrl Pts',(0.0892318011706237,1.33489254525337,
0.416863803530356));
#16358=CARTESIAN_POINT('Ctrl Pts',(0.100088380073201,1.32404321751407,0.624288602298589));
#16359=CARTESIAN_POINT('Ctrl Pts',(0.212439875011655,1.41741816253371,-0.00240566592686199));
#16360=CARTESIAN_POINT('Ctrl Pts',(0.223274062163905,1.40657840226088,0.20502076110302));
#16361=CARTESIAN_POINT('Ctrl Pts',(0.234108278795672,1.39573903465802,0.412447205628077));
#16362=CARTESIAN_POINT('Ctrl Pts',(0.244942059060342,1.38489960928785,0.619873667633733));
#16363=CARTESIAN_POINT('Ctrl Pts',(0.276041299849618,1.42253242682652,-0.00547191373834488));
#16364=CARTESIAN_POINT('Ctrl Pts',(0.286868655882245,1.41170146982041,0.201955326984501));
#16365=CARTESIAN_POINT('Ctrl Pts',(0.297695769965166,1.40087072543886,0.409382589539965));
#16366=CARTESIAN_POINT('Ctrl Pts',(0.308522637995069,1.39004019713626,0.616809874278785));
#16367=CARTESIAN_POINT('Ctrl Pts',(2.26869304592592E-17,1.12356026268968,
-3.16587034365767E-17));
#16368=CARTESIAN_POINT('Ctrl Pts',(0.0107558363321878,1.11284719399672,
0.205233583245308));
#16369=CARTESIAN_POINT('Ctrl Pts',(0.0215116733095221,1.10213436178043,
0.410467178800746));
#16370=CARTESIAN_POINT('Ctrl Pts',(0.0322675109428289,1.09142177001972,
0.615700786872884));
#16371=CARTESIAN_POINT('Ctrl Pts',(0.308522637995069,1.39004019713626,0.616809874278785));
#16372=CARTESIAN_POINT('Ctrl Pts',(0.297790973931072,1.40077548928706,0.411206561171438));
#16373=CARTESIAN_POINT('Ctrl Pts',(0.287059068122271,1.41151099373341,0.205603269859031));
#16374=CARTESIAN_POINT('Ctrl Pts',(0.276326924564681,1.42224670711126,-2.68882138776405E-16));
#16375=CARTESIAN_POINT('Ctrl Pts',(10.5166159648474,-1.4155315881283,0.));
#16376=CARTESIAN_POINT('Ctrl Pts',(10.5064062201588,-1.40475637621136,0.205603291426271));
#16377=CARTESIAN_POINT('Ctrl Pts',(10.4961964754701,-1.39398116429443,0.411206582852543));
#16378=CARTESIAN_POINT('Ctrl Pts',(10.4859867307814,-1.38320595237749,0.616809874278814));
#16379=CARTESIAN_POINT('Ctrl Pts',(7.10318628475318,-1.599994843061,0.));
#16380=CARTESIAN_POINT('Ctrl Pts',(7.09978773046573,-1.58921963114407,0.205603291426271));
#16381=CARTESIAN_POINT('Ctrl Pts',(7.09638917617828,-1.57844441922713,0.411206582852543));
#16382=CARTESIAN_POINT('Ctrl Pts',(7.09299062189083,-1.5676692073102,0.616809874278814));
#16383=CARTESIAN_POINT('Ctrl Pts',(3.68975660465893,-1.68747752195839,0.));
#16384=CARTESIAN_POINT('Ctrl Pts',(3.69316924077269,-1.67670231004145,0.205603291426272));
#16385=CARTESIAN_POINT('Ctrl Pts',(3.69658187688646,-1.66592709812452,0.411206582852543));
#16386=CARTESIAN_POINT('Ctrl Pts',(3.69999451300023,-1.65515188620758,0.616809874278814));
#16387=CARTESIAN_POINT('Ctrl Pts',(0.276326924564679,-1.42224670711126,
0.));
#16388=CARTESIAN_POINT('Ctrl Pts',(0.286550751079662,-1.41147149519433,
0.205603291426271));
#16389=CARTESIAN_POINT('Ctrl Pts',(0.296774577594646,-1.40069628327739,
0.411206582852543));
#16390=CARTESIAN_POINT('Ctrl Pts',(0.306998404109629,-1.38992107136046,
0.616809874278814));
#16391=CARTESIAN_POINT('Origin',(0.,-1.4,0.));
#16392=CARTESIAN_POINT('Origin',(5.4,-8.13935059369636E-18,0.9));
#16393=CARTESIAN_POINT('Ctrl Pts',(0.276326924564679,1.42224670711126,0.));
#16394=CARTESIAN_POINT('Ctrl Pts',(0.286550751079662,1.41147149519433,0.205603291426271));
#16395=CARTESIAN_POINT('Ctrl Pts',(0.296774577594645,1.40069628327739,0.411206582852543));
#16396=CARTESIAN_POINT('Ctrl Pts',(0.306998404109628,1.38992107136046,0.616809874278814));
#16397=CARTESIAN_POINT('Ctrl Pts',(3.68975660465893,1.68747752195839,0.));
#16398=CARTESIAN_POINT('Ctrl Pts',(3.6931692407727,1.67670231004145,0.205603291426271));
#16399=CARTESIAN_POINT('Ctrl Pts',(3.69658187688646,1.66592709812452,0.411206582852543));
#16400=CARTESIAN_POINT('Ctrl Pts',(3.69999451300023,1.65515188620758,0.616809874278814));
#16401=CARTESIAN_POINT('Ctrl Pts',(7.10318628475318,1.599994843061,0.));
#16402=CARTESIAN_POINT('Ctrl Pts',(7.09978773046573,1.58921963114407,0.205603291426271));
#16403=CARTESIAN_POINT('Ctrl Pts',(7.09638917617828,1.57844441922713,0.411206582852543));
#16404=CARTESIAN_POINT('Ctrl Pts',(7.09299062189083,1.5676692073102,0.616809874278814));
#16405=CARTESIAN_POINT('Ctrl Pts',(10.5166159648474,1.4155315881283,0.));
#16406=CARTESIAN_POINT('Ctrl Pts',(10.5064062201588,1.40475637621136,0.205603291426271));
#16407=CARTESIAN_POINT('Ctrl Pts',(10.4961964754701,1.39398116429443,0.411206582852543));
#16408=CARTESIAN_POINT('Ctrl Pts',(10.4859867307814,1.38320595237749,0.616809874278814));
#16409=CARTESIAN_POINT('Origin',(10.8,1.4,0.));
#22112=UNCERTAINTY_MEASURE_WITH_UNIT(LENGTH_MEASURE(0.001),#22130,
'DISTANCE_ACCURACY_VALUE',
'Maximum model space distance between geometric entities at asserted c
onnectivities');
#22117=UNCERTAINTY_MEASURE_WITH_UNIT(LENGTH_MEASURE(0.001),#22130,
'DISTANCE_ACCURACY_VALUE',
'Maximum model space distance between geometric entities at asserted c
onnectivities');
#22124=(
GEOMETRIC_REPRESENTATION_CONTEXT(3)
GLOBAL_UNCERTAINTY_ASSIGNED_CONTEXT((#22112))
GLOBAL_UNIT_ASSIGNED_CONTEXT((#22130,#22132,#22133))
REPRESENTATION_CONTEXT('','3D')
);
#22129=(
GEOMETRIC_REPRESENTATION_CONTEXT(3)
GLOBAL_UNCERTAINTY_ASSIGNED_CONTEXT((#22117))
GLOBAL_UNIT_ASSIGNED_CONTEXT((#22130,#22132,#22133))
REPRESENTATION_CONTEXT('','3D')
);
#22130=(
LENGTH_UNIT()
NAMED_UNIT(*)
SI_UNIT(.CENTI.,.METRE.)
);
#22132=(
NAMED_UNIT(*)
PLANE_ANGLE_UNIT()
SI_UNIT($,.RADIAN.)
);
#22133=(
NAMED_UNIT(*)
SI_UNIT($,.STERADIAN.)
SOLID_ANGLE_UNIT()
);
#22140=SHAPE_DEFINITION_REPRESENTATION(#22151,#22178);
#22151=PRODUCT_DEFINITION_SHAPE('',$,#22190);
#22178=SHAPE_REPRESENTATION('',(#9198),#22124);
#22183=PRODUCT_DEFINITION_CONTEXT('part definition',#22218,'design');
#22190=PRODUCT_DEFINITION('2026-11-10-05-10-49-236',
'Lower structural shell',#22201,#22183);
#22201=PRODUCT_DEFINITION_FORMATION('',$,#22226);
#22218=APPLICATION_CONTEXT(
'Core Data for Automotive Mechanical Design Process');
#22219=PRODUCT_CONTEXT('part definition',#22218,'mechanical');
#22226=PRODUCT('2026-11-10-05-10-49-236','Lower structural shell',$,(#22219));
#22235=PRESENTATION_STYLE_ASSIGNMENT((#22243));
#22243=SURFACE_STYLE_USAGE(.BOTH.,#22251);
#22251=SURFACE_SIDE_STYLE('',(#22259));
#22259=SURFACE_STYLE_FILL_AREA(#22267);
#22267=FILL_AREA_STYLE('Structural dark blue',(#22275));
#22275=FILL_AREA_STYLE_COLOUR('Structural dark blue',#22283);
#22283=COLOUR_RGB('Structural dark blue',0.0901960784313725,0.270588235294118,
0.513725490196078);
ENDSEC;
END-ISO-10303-21;
